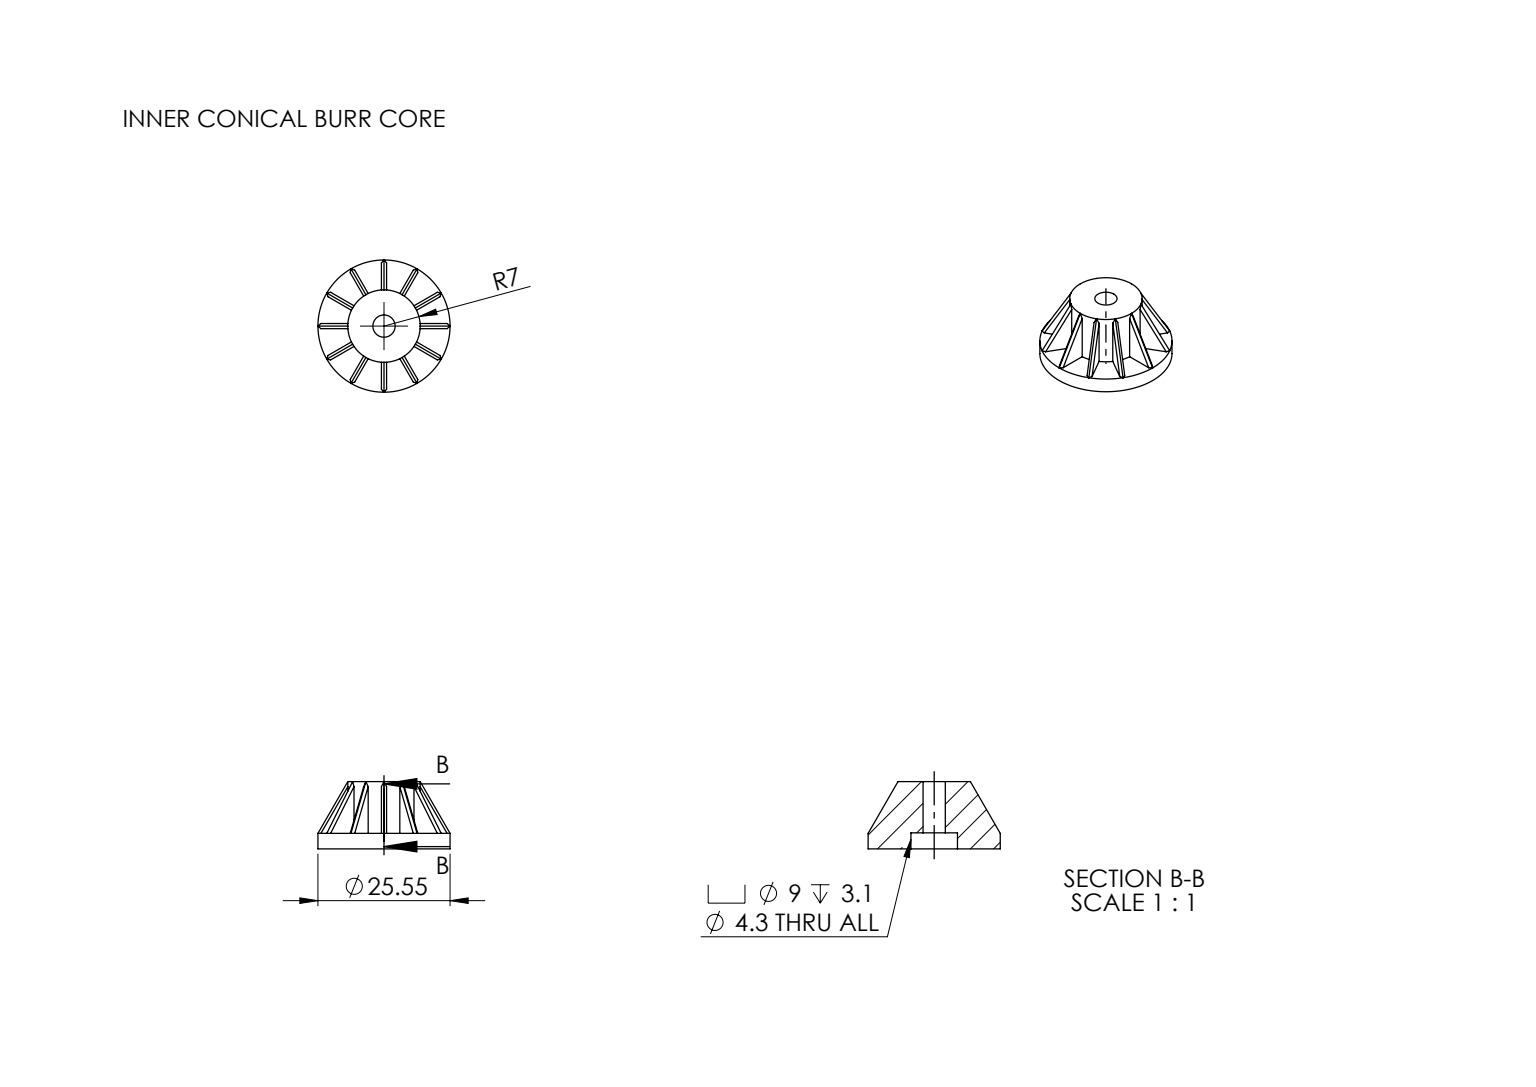
ISO-10303-21;
HEADER;
FILE_DESCRIPTION (('STEP AP214'),
    '1' );
FILE_NAME ('Inner Conical Burr Core.step',
    '2026-10-04T07:23:31',
    ( '' ),
    ( '' ),
    'SwSTEP 2.0',
    'SolidWorks 2026',
    '' );
FILE_SCHEMA (( 'AUTOMOTIVE_DESIGN' ));
ENDSEC;

DATA;
#8=VECTOR ( 'NONE', #4080, 1000.000000000000114 ) ;
#13=CARTESIAN_POINT ( 'NONE',  ( 6.296693311223917178, 19.03096903053430822, -3.058047309049999996 ) ) ;
#14=PRODUCT_DEFINITION ( 'UNKNOWN', '', #3514, #8030 ) ;
#17=EDGE_LOOP ( 'NONE', ( #5267, #4224, #10502 ) ) ;
#18=ORIENTED_EDGE ( 'NONE', *, *, #6824, .T. ) ;
#20=VERTEX_POINT ( 'NONE', #2725 ) ;
#21=DIRECTION ( 'NONE',  ( -0.000000000000000000, 1.000000000000000000, -0.000000000000000000 ) ) ;
#22=EDGE_LOOP ( 'NONE', ( #2895, #8859 ) ) ;
#23=FACE_OUTER_BOUND ( 'NONE', #10644, .T. ) ;
#26=EDGE_CURVE ( 'NONE', #5713, #6934, #4532, .T. ) ;
#34=AXIS2_PLACEMENT_3D ( 'NONE', #3449, #3389, #7599 ) ;
#41=LINE ( 'NONE', #2461, #2290 ) ;
#45=EDGE_CURVE ( 'NONE', #4079, #9358, #1978, .T. ) ;
#49=VECTOR ( 'NONE', #6901, 1000.000000000000000 ) ;
#53=LINE ( 'NONE', #1004, #7949 ) ;
#54=VECTOR ( 'NONE', #4758, 1000.000000000000000 ) ;
#62=DIRECTION ( 'NONE',  ( 0.000000000000000000, 1.000000000000000000, 0.000000000000000000 ) ) ;
#63=PLANE ( 'NONE',  #9863 ) ;
#78=CARTESIAN_POINT ( 'NONE',  ( 3.785909150703048454, 19.34316356887877220, -5.890223162633865250 ) ) ;
#89=CARTESIAN_POINT ( 'NONE',  ( 6.999999999999997335, 19.66631150450990617, 0.1668442477450632899 ) ) ;
#102=ORIENTED_EDGE ( 'NONE', *, *, #949, .F. ) ;
#115=CARTESIAN_POINT ( 'NONE',  ( 0.000000000000000000, 20.00000000000000355, 0.000000000000000000 ) ) ;
#136=CARTESIAN_POINT ( 'NONE',  ( -7.211537444790369733, 10.00000000000000355, -6.776463540776874517 ) ) ;
#144=ADVANCED_FACE ( 'NONE', ( #9538 ), #8711, .T. ) ;
#150=CYLINDRICAL_SURFACE ( 'NONE', #10591, 4.500000000000000888 ) ;
#151=DIRECTION ( 'NONE',  ( -0.8838834764831844382, -0.3535533905932726206, 0.3061862178478983454 ) ) ;
#153=AXIS2_PLACEMENT_3D ( 'NONE', #2387, #10130, #10796 ) ;
#154=CIRCLE ( 'NONE', #1379, 12.77350269189627063 ) ;
#159=CARTESIAN_POINT ( 'NONE',  ( -6.062177826491028654, 20.00000000000000355, -3.500000000000069722 ) ) ;
#162=CARTESIAN_POINT ( 'NONE',  ( -3.066987298107830995, 10.00000000000000355, 6.312177826491043753 ) ) ;
#165=CARTESIAN_POINT ( 'NONE',  ( 4.500000000000000888, 10.10000000000000497, 0.000000000000000000 ) ) ;
#173=CARTESIAN_POINT ( 'NONE',  ( 2.632990618166809235E-16, 7.000000000000003553, 2.149999999999999911 ) ) ;
#174=DIRECTION ( 'NONE',  ( 0.000000000000000000, 0.000000000000000000, 1.000000000000000000 ) ) ;
#185=DIRECTION ( 'NONE',  ( 0.000000000000000000, -1.000000000000000000, 0.000000000000000000 ) ) ;
#196=EDGE_CURVE ( 'NONE', #620, #978, #10271, .T. ) ;
#200=ORIENTED_EDGE ( 'NONE', *, *, #382, .F. ) ;
#213=ORIENTED_EDGE ( 'NONE', *, *, #10024, .F. ) ;
#219=EDGE_LOOP ( 'NONE', ( #2618, #7161, #8269, #2550 ) ) ;
#221=CARTESIAN_POINT ( 'NONE',  ( 0.000000000000000000, 7.000000000000003553, 0.000000000000000000 ) ) ;
#222=DIRECTION ( 'NONE',  ( 0.000000000000000000, 1.000000000000000000, 0.000000000000000000 ) ) ;
#244=DIRECTION ( 'NONE',  ( 0.000000000000000000, 1.000000000000000000, 0.000000000000000000 ) ) ;
#253=AXIS2_PLACEMENT_3D ( 'NONE', #6290, #1159, #5410 ) ;
#263=DIRECTION ( 'NONE',  ( 0.6546536707079723127, -0.000000000000000000, -0.7559289460184587250 ) ) ;
#276=( BOUNDED_CURVE ( )  B_SPLINE_CURVE ( 3, ( #9723, #2251, #5583, #2149 ),
 .UNSPECIFIED., .F., .F. ) 
 B_SPLINE_CURVE_WITH_KNOTS ( ( 4, 4 ),
 ( 2.284520705739658375, 2.356010155625179792 ),
 .UNSPECIFIED. ) 
 CURVE ( )  GEOMETRIC_REPRESENTATION_ITEM ( )  RATIONAL_B_SPLINE_CURVE ( ( 1.000000000000000000, 0.9995741502243209453, 0.9995741502243209453, 1.000000000000000000 ) ) 
 REPRESENTATION_ITEM ( '' )  );
#277=DIRECTION ( 'NONE',  ( -0.2500000000000041078, -0.8660254037844380415, 0.4330127018922181881 ) ) ;
#280=DIRECTION ( 'NONE',  ( -0.000000000000000000, 1.000000000000000000, -0.000000000000000000 ) ) ;
#281=CARTESIAN_POINT ( 'NONE',  ( -0.5000000000000001110, 10.00000000000000355, -6.982120021884469452 ) ) ;
#283=DIRECTION ( 'NONE',  ( 0.000000000000000000, 0.000000000000000000, 1.000000000000000000 ) ) ;
#287=PLANE ( 'NONE',  #10755 ) ;
#291=ORIENTED_EDGE ( 'NONE', *, *, #10657, .F. ) ;
#294=ORIENTED_EDGE ( 'NONE', *, *, #5471, .F. ) ;
#301=CARTESIAN_POINT ( 'NONE',  ( -5.978755702618581580, 19.66631150450990617, 3.644491357022453748 ) ) ;
#302=CARTESIAN_POINT ( 'NONE',  ( 0.2500000000000019984, 0.000000000000000000, -0.4330127018922181326 ) ) ;
#307=EDGE_CURVE ( 'NONE', #620, #1515, #1911, .T. ) ;
#308=DIRECTION ( 'NONE',  ( 0.000000000000000000, 1.000000000000000000, 0.000000000000000000 ) ) ;
#309=ADVANCED_FACE ( 'NONE', ( #3677 ), #6334, .F. ) ;
#312=CARTESIAN_POINT ( 'NONE',  ( 11.42163336986832611, 7.781088913245561400, -7.171633369868279928 ) ) ;
#320=AXIS2_PLACEMENT_3D ( 'NONE', #10601, #7911, #7226 ) ;
#324=CARTESIAN_POINT ( 'NONE',  ( -5.812177826491105037, 10.00000000000000355, 3.933012701892163676 ) ) ;
#328=AXIS2_PLACEMENT_3D ( 'NONE', #8665, #3636, #7020 ) ;
#334=( BOUNDED_CURVE ( )  B_SPLINE_CURVE ( 3, ( #9140, #1571, #4960, #8309 ),
 .UNSPECIFIED., .F., .F. ) 
 B_SPLINE_CURVE_WITH_KNOTS ( ( 4, 4 ),
 ( 2.284520705739657931, 2.356010155625178015 ),
 .UNSPECIFIED. ) 
 CURVE ( )  GEOMETRIC_REPRESENTATION_ITEM ( )  RATIONAL_B_SPLINE_CURVE ( ( 1.000000000000000000, 0.9995741502243209453, 0.9995741502243209453, 1.000000000000000000 ) ) 
 REPRESENTATION_ITEM ( '' )  );
#336=DIRECTION ( 'NONE',  ( 0.000000000000000000, 0.000000000000000000, -1.000000000000000000 ) ) ;
#340=ORIENTED_EDGE ( 'NONE', *, *, #4019, .T. ) ;
#343=CYLINDRICAL_SURFACE ( 'NONE', #9212, 12.77350269189627063 ) ;
#354=CARTESIAN_POINT ( 'NONE',  ( 6.145599950363597408, 19.66631150450990972, -3.355508642977475198 ) ) ;
#363=AXIS2_PLACEMENT_3D ( 'NONE', #7383, #10762, #7726 ) ;
#370=CARTESIAN_POINT ( 'NONE',  ( -4.336808689942017736E-16, 20.00000000000000355, 6.999999999999997335 ) ) ;
#375=VERTEX_POINT ( 'NONE', #4612 ) ;
#378=CARTESIAN_POINT ( 'NONE',  ( -7.171633369868398056, 7.781088913245559624, 11.42163336986824973 ) ) ;
#382=EDGE_CURVE ( 'NONE', #8258, #528, #7233, .T. ) ;
#384=AXIS2_PLACEMENT_3D ( 'NONE', #4121, #4890, #851 ) ;
#386=CARTESIAN_POINT ( 'NONE',  ( -5.796693311223947376, 10.00000000000000355, 3.924072712834399734 ) ) ;
#396=EDGE_CURVE ( 'NONE', #5862, #7391, #2207, .T. ) ;
#397=CIRCLE ( 'NONE', #8311, 6.999999999999997335 ) ;
#399=VERTEX_POINT ( 'NONE', #8842 ) ;
#401=CIRCLE ( 'NONE', #10807, 6.999999999999997335 ) ;
#403=CARTESIAN_POINT ( 'NONE',  ( 0.000000000000000000, 20.00000000000000355, -6.999999999999997335 ) ) ;
#417=VERTEX_POINT ( 'NONE', #2913 ) ;
#423=CARTESIAN_POINT ( 'NONE',  ( -2.857142857142858983, 10.00000000000000355, -9.474358296526935064 ) ) ;
#425=FACE_OUTER_BOUND ( 'NONE', #10415, .T. ) ;
#426=PLANE ( 'NONE',  #3198 ) ;
#428=EDGE_LOOP ( 'NONE', ( #6689, #3315, #4054 ) ) ;
#429=ORIENTED_EDGE ( 'NONE', *, *, #6271, .F. ) ;
#430=ORIENTED_EDGE ( 'NONE', *, *, #4396, .T. ) ;
#432=DIRECTION ( 'NONE',  ( -0.4999999999999919509, 0.000000000000000000, -0.8660254037844432595 ) ) ;
#438=ORIENTED_EDGE ( 'NONE', *, *, #10019, .T. ) ;
#446=EDGE_CURVE ( 'NONE', #7282, #1433, #4666, .T. ) ;
#447=CARTESIAN_POINT ( 'NONE',  ( 0.000000000000000000, 20.00000000000000355, 0.000000000000000000 ) ) ;
#453=EDGE_CURVE ( 'NONE', #3864, #1133, #3229, .T. ) ;
#462=PLANE ( 'NONE',  #6027 ) ;
#472=CARTESIAN_POINT ( 'NONE',  ( 0.000000000000000000, 20.00000000000000355, 0.000000000000000000 ) ) ;
#473=CARTESIAN_POINT ( 'NONE',  ( -6.348076211353412823, 10.00000000000000355, 11.26313972081436532 ) ) ;
#478=EDGE_CURVE ( 'NONE', #10364, #8941, #3461, .T. ) ;
#496=ORIENTED_EDGE ( 'NONE', *, *, #2584, .T. ) ;
#501=ORIENTED_EDGE ( 'NONE', *, *, #4410, .F. ) ;
#512=LINE ( 'NONE', #7202, #5833 ) ;
#523=CARTESIAN_POINT ( 'NONE',  ( 5.446152422706636465, 10.00000000000000355, -2.566987298107767490 ) ) ;
#524=ORIENTED_EDGE ( 'NONE', *, *, #1672, .T. ) ;
#525=EDGE_CURVE ( 'NONE', #5936, #10248, #7856, .T. ) ;
#526=CIRCLE ( 'NONE', #1771, 12.77350269189627063 ) ;
#528=VERTEX_POINT ( 'NONE', #281 ) ;
#531=LINE ( 'NONE', #8048, #2356 ) ;
#557=CARTESIAN_POINT ( 'NONE',  ( -6.999999999999994671, 19.66631150450992749, -0.1668442477451158867 ) ) ;
#566=AXIS2_PLACEMENT_3D ( 'NONE', #6788, #151, #987 ) ;
#567=EDGE_CURVE ( 'NONE', #9293, #10413, #10782, .T. ) ;
#569=AXIS2_PLACEMENT_3D ( 'NONE', #4292, #5896, #6784 ) ;
#570=DIRECTION ( 'NONE',  ( -1.000000000000000000, 0.000000000000000000, 0.000000000000000000 ) ) ;
#573=CARTESIAN_POINT ( 'NONE',  ( 3.058047309050023088, 10.00000000000000355, -6.296693311223907408 ) ) ;
#576=AXIS2_PLACEMENT_3D ( 'NONE', #6748, #5973, #10110 ) ;
#583=CIRCLE ( 'NONE', #4834, 6.999999999999997335 ) ;
#586=ORIENTED_EDGE ( 'NONE', *, *, #567, .T. ) ;
#588=DIRECTION ( 'NONE',  ( -1.000000000000000000, 0.000000000000000000, -1.047444401652940007E-14 ) ) ;
#592=PLANE ( 'NONE',  #2028 ) ;
#593=DIRECTION ( 'NONE',  ( -0.000000000000000000, -1.000000000000000000, -0.000000000000000000 ) ) ;
#594=DIRECTION ( 'NONE',  ( 0.000000000000000000, 1.000000000000000000, 0.000000000000000000 ) ) ;
#595=AXIS2_PLACEMENT_3D ( 'NONE', #2399, #9367, #7543 ) ;
#600=CARTESIAN_POINT ( 'NONE',  ( -3.924072712834378862, 19.03096903053431888, -5.796693311223959810 ) ) ;
#603=ORIENTED_EDGE ( 'NONE', *, *, #8062, .F. ) ;
#604=LINE ( 'NONE', #4915, #6711 ) ;
#606=LINE ( 'NONE', #10829, #1633 ) ;
#613=LINE ( 'NONE', #784, #5147 ) ;
#615=PLANE ( 'NONE',  #10718 ) ;
#617=DIRECTION ( 'NONE',  ( -0.5000000000000009992, -0.8660254037844380415, -5.237222008264710288E-15 ) ) ;
#620=VERTEX_POINT ( 'NONE', #910 ) ;
#622=ORIENTED_EDGE ( 'NONE', *, *, #2384, .T. ) ;
#623=UNCERTAINTY_MEASURE_WITH_UNIT (LENGTH_MEASURE( 1.000000000000000082E-05 ), #723, 'distance_accuracy_value', 'NONE');
#626=CARTESIAN_POINT ( 'NONE',  ( 6.296693311223917178, 10.00000000000000355, -3.058047309050000440 ) ) ;
#628=ADVANCED_FACE ( 'NONE', ( #4398 ), #5994, .T. ) ;
#639=CARTESIAN_POINT ( 'NONE',  ( -3.644491357022560329, 19.66631150450991328, 5.978755702618518519 ) ) ;
#643=ADVANCED_FACE ( 'NONE', ( #9413 ), #7049, .T. ) ;
#656=ORIENTED_EDGE ( 'NONE', *, *, #8957, .F. ) ;
#660=EDGE_LOOP ( 'NONE', ( #8805, #3492, #5444 ) ) ;
#664=VECTOR ( 'NONE', #5477, 1000.000000000000000 ) ;
#667=( NAMED_UNIT ( * ) SI_UNIT ( $, .STERADIAN. ) SOLID_ANGLE_UNIT ( ) );
#671=DIRECTION ( 'NONE',  ( -0.5000000000000009992, -0.8660254037844380415, -5.237222008264710288E-15 ) ) ;
#673=APPLICATION_CONTEXT ( 'automotive_design' ) ;
#680=( BOUNDED_CURVE ( )  B_SPLINE_CURVE ( 3, ( #1827, #826, #9316, #8327 ),
 .UNSPECIFIED., .F., .F. ) 
 B_SPLINE_CURVE_WITH_KNOTS ( ( 4, 4 ),
 ( 2.284520705739662816, 2.356010155625183344 ),
 .UNSPECIFIED. ) 
 CURVE ( )  GEOMETRIC_REPRESENTATION_ITEM ( )  RATIONAL_B_SPLINE_CURVE ( ( 1.000000000000000000, 0.9995741502243209453, 0.9995741502243209453, 1.000000000000000000 ) ) 
 REPRESENTATION_ITEM ( '' )  );
#685=FACE_OUTER_BOUND ( 'NONE', #2794, .T. ) ;
#688=EDGE_CURVE ( 'NONE', #7766, #10229, #10434, .T. ) ;
#689=VERTEX_POINT ( 'NONE', #7976 ) ;
#691=PLANE ( 'NONE',  #569 ) ;
#692=CARTESIAN_POINT ( 'NONE',  ( 5.796693311223918066, 10.00000000000000355, -3.924072712834439702 ) ) ;
#694=DIRECTION ( 'NONE',  ( 0.5000000000000009992, 0.8660254037844380415, 5.237222008264710288E-15 ) ) ;
#699=EDGE_CURVE ( 'NONE', #8354, #9358, #9835, .T. ) ;
#701=LINE ( 'NONE', #1368, #8 ) ;
#723=( LENGTH_UNIT ( ) NAMED_UNIT ( * ) SI_UNIT ( .MILLI., .METRE. ) );
#726=CARTESIAN_POINT ( 'NONE',  ( 0.000000000000000000, 10.00000000000000355, 0.000000000000000000 ) ) ;
#731=ORIENTED_EDGE ( 'NONE', *, *, #3404, .F. ) ;
#732=ORIENTED_EDGE ( 'NONE', *, *, #949, .T. ) ;
#737=LINE ( 'NONE', #6601, #10727 ) ;
#740=CARTESIAN_POINT ( 'NONE',  ( -2.850480947161592393, 19.75000000000000000, -5.937177826491103261 ) ) ;
#742=FACE_OUTER_BOUND ( 'NONE', #10182, .T. ) ;
#748=VERTEX_POINT ( 'NONE', #2062 ) ;
#757=CARTESIAN_POINT ( 'NONE',  ( 3.924072712834419718, 10.00000000000000355, 5.796693311223933165 ) ) ;
#758=AXIS2_PLACEMENT_3D ( 'NONE', #2810, #6208, #9567 ) ;
#760=ORIENTED_EDGE ( 'NONE', *, *, #1166, .T. ) ;
#761=VECTOR ( 'NONE', #8157, 1000.000000000000000 ) ;
#762=VECTOR ( 'NONE', #6178, 1000.000000000000114 ) ;
#768=LINE ( 'NONE', #8263, #2119 ) ;
#772=FACE_OUTER_BOUND ( 'NONE', #7291, .T. ) ;
#773=CARTESIAN_POINT ( 'NONE',  ( 0.000000000000000000, 7.000000000000003553, -4.500000000000000888 ) ) ;
#775=CIRCLE ( 'NONE', #8006, 6.999999999999997335 ) ;
#776=EDGE_LOOP ( 'NONE', ( #10832, #8415, #8860, #10571 ) ) ;
#777=EDGE_LOOP ( 'NONE', ( #3949, #5123, #7353, #340, #8376, #4998 ) ) ;
#784=CARTESIAN_POINT ( 'NONE',  ( -5.437177826491026877, 19.75000000000000355, -3.716506350946172876 ) ) ;
#793=ORIENTED_EDGE ( 'NONE', *, *, #8651, .F. ) ;
#797=EDGE_CURVE ( 'NONE', #6584, #9935, #4622, .T. ) ;
#801=LINE ( 'NONE', #740, #2804 ) ;
#805=PLANE ( 'NONE',  #10636 ) ;
#808=ORIENTED_EDGE ( 'NONE', *, *, #2666, .F. ) ;
#812=EDGE_CURVE ( 'NONE', #8587, #10544, #2924, .T. ) ;
#816=DIRECTION ( 'NONE',  ( 0.8838834764831839941, 0.3535533905932757293, 0.3061862178478963470 ) ) ;
#817=DIRECTION ( 'NONE',  ( 0.7559289460184611675, 0.000000000000000000, -0.6546536707079694262 ) ) ;
#818=ADVANCED_FACE ( 'NONE', ( #6639 ), #615, .F. ) ;
#819=ORIENTED_EDGE ( 'NONE', *, *, #6227, .T. ) ;
#824=VERTEX_POINT ( 'NONE', #3298 ) ;
#826=CARTESIAN_POINT ( 'NONE',  ( -3.644491357022439537, 19.66631150450991328, -5.978755702618592238 ) ) ;
#827=DIRECTION ( 'NONE',  ( -0.3061862178479081154, 0.3535533905932724541, 0.8838834764831812185 ) ) ;
#829=ORIENTED_EDGE ( 'NONE', *, *, #10797, .T. ) ;
#842=ORIENTED_EDGE ( 'NONE', *, *, #8332, .T. ) ;
#851=DIRECTION ( 'NONE',  ( 0.000000000000000000, 0.000000000000000000, 1.000000000000000000 ) ) ;
#854=FACE_OUTER_BOUND ( 'NONE', #4694, .T. ) ;
#858=ORIENTED_EDGE ( 'NONE', *, *, #9260, .F. ) ;
#863=CARTESIAN_POINT ( 'NONE',  ( 3.058047309049977791, 19.03096903053433309, 6.296693311223928724 ) ) ;
#871=LINE ( 'NONE', #3396, #9310 ) ;
#874=DIRECTION ( 'NONE',  ( -0.000000000000000000, -1.000000000000000000, -0.000000000000000000 ) ) ;
#880=VECTOR ( 'NONE', #1605, 1000.000000000000114 ) ;
#895=DIRECTION ( 'NONE',  ( -0.1767766952966370597, -0.3535533905932738419, 0.9185586535436917055 ) ) ;
#897=CYLINDRICAL_SURFACE ( 'NONE', #5644, 6.999999999999997335 ) ;
#903=DIRECTION ( 'NONE',  ( 0.000000000000000000, 0.000000000000000000, 1.000000000000000000 ) ) ;
#909=ORIENTED_EDGE ( 'NONE', *, *, #4582, .F. ) ;
#910=CARTESIAN_POINT ( 'NONE',  ( -3.500000000000049294, 20.00000000000000355, 6.062177826491040200 ) ) ;
#915=VERTEX_POINT ( 'NONE', #4880 ) ;
#925=CARTESIAN_POINT ( 'NONE',  ( 6.982120021884465899, 19.03096903053429401, 0.5000000000000244249 ) ) ;
#938=LINE ( 'NONE', #4306, #3108 ) ;
#943=CIRCLE ( 'NONE', #10817, 2.149999999999999911 ) ;
#947=AXIS2_PLACEMENT_3D ( 'NONE', #8244, #10531, #8975 ) ;
#949=EDGE_CURVE ( 'NONE', #3818, #3051, #10896, .T. ) ;
#964=VECTOR ( 'NONE', #1264, 1000.000000000000000 ) ;
#967=ORIENTED_EDGE ( 'NONE', *, *, #2281, .F. ) ;
#978=VERTEX_POINT ( 'NONE', #1668 ) ;
#979=CARTESIAN_POINT ( 'NONE',  ( 0.000000000000000000, 10.00000000000000355, 0.000000000000000000 ) ) ;
#984=( BOUNDED_CURVE ( )  B_SPLINE_CURVE ( 3, ( #8489, #6736, #6844, #2563 ),
 .UNSPECIFIED., .F., .T. ) 
 B_SPLINE_CURVE_WITH_KNOTS ( ( 4, 4 ),
 ( 3.927175151554402888, 3.998664601439924304 ),
 .UNSPECIFIED. ) 
 CURVE ( )  GEOMETRIC_REPRESENTATION_ITEM ( )  RATIONAL_B_SPLINE_CURVE ( ( 1.000000000000000000, 0.9995741502243209453, 0.9995741502243209453, 1.000000000000000000 ) ) 
 REPRESENTATION_ITEM ( '' )  );
#986=LINE ( 'NONE', #9545, #1256 ) ;
#987=DIRECTION ( 'NONE',  ( -0.4330127018922191318, 0.8660254037844380415, -0.2500000000000026090 ) ) ;
#988=DIRECTION ( 'NONE',  ( 0.4999999999999980016, 0.000000000000000000, 0.8660254037844398178 ) ) ;
#990=ORIENTED_EDGE ( 'NONE', *, *, #7446, .T. ) ;
#992=LINE ( 'NONE', #3335, #8666 ) ;
#996=ORIENTED_EDGE ( 'NONE', *, *, #453, .F. ) ;
#997=EDGE_CURVE ( 'NONE', #6764, #7282, #10390, .T. ) ;
#999=DIRECTION ( 'NONE',  ( 0.000000000000000000, -1.000000000000000000, 0.000000000000000000 ) ) ;
#1001=ADVANCED_FACE ( 'NONE', ( #1013 ), #7805, .F. ) ;
#1004=CARTESIAN_POINT ( 'NONE',  ( -11.06217782649114412, 10.00000000000000533, 6.386751345948026071 ) ) ;
#1008=EDGE_CURVE ( 'NONE', #9883, #7303, #1839, .T. ) ;
#1013=FACE_OUTER_BOUND ( 'NONE', #2172, .T. ) ;
#1016=EDGE_CURVE ( 'NONE', #8941, #10020, #1128, .T. ) ;
#1017=ORIENTED_EDGE ( 'NONE', *, *, #3787, .T. ) ;
#1019=( GEOMETRIC_REPRESENTATION_CONTEXT ( 3 ) GLOBAL_UNCERTAINTY_ASSIGNED_CONTEXT ( ( #1395 ) ) GLOBAL_UNIT_ASSIGNED_CONTEXT ( ( #2530, #3296, #4932 ) ) REPRESENTATION_CONTEXT ( 'NONE', 'WORKASPACE' ) );
#1026=CARTESIAN_POINT ( 'NONE',  ( -5.890223162633902554, 19.34316356887877220, 3.785909150702991166 ) ) ;
#1032=EDGE_LOOP ( 'NONE', ( #3309, #9854, #6146, #10751, #8965, #2173 ) ) ;
#1037=VECTOR ( 'NONE', #2963, 1000.000000000000000 ) ;
#1043=DIRECTION ( 'NONE',  ( -0.2499999999999980016, 0.8660254037844380415, -0.4330127018922217408 ) ) ;
#1049=ORIENTED_EDGE ( 'NONE', *, *, #196, .T. ) ;
#1068=DIRECTION ( 'NONE',  ( 0.000000000000000000, 0.000000000000000000, -1.000000000000000000 ) ) ;
#1069=DIRECTION ( 'NONE',  ( 0.5000000000000009992, 0.000000000000000000, -0.8660254037844380415 ) ) ;
#1071=AXIS2_PLACEMENT_3D ( 'NONE', #8171, #7438, #3226 ) ;
#1073=AXIS2_PLACEMENT_3D ( 'NONE', #10856, #9237, #8408 ) ;
#1074=ORIENTED_EDGE ( 'NONE', *, *, #3776, .T. ) ;
#1079=LINE ( 'NONE', #10349, #6951 ) ;
#1091=ORIENTED_EDGE ( 'NONE', *, *, #2592, .F. ) ;
#1092=ORIENTED_EDGE ( 'NONE', *, *, #10848, .F. ) ;
#1101=CARTESIAN_POINT ( 'NONE',  ( 0.000000000000000000, 7.000000000000003553, 0.000000000000000000 ) ) ;
#1102=FACE_OUTER_BOUND ( 'NONE', #9137, .T. ) ;
#1104=VECTOR ( 'NONE', #7309, 999.9999999999998863 ) ;
#1107=CARTESIAN_POINT ( 'NONE',  ( 0.5000000000000000000, 0.000000000000000000, 0.000000000000000000 ) ) ;
#1109=CIRCLE ( 'NONE', #2847, 6.999999999999997335 ) ;
#1112=CARTESIAN_POINT ( 'NONE',  ( 5.796693311223892309, 19.03096903053431532, 3.924072712834481447 ) ) ;
#1117=( BOUNDED_CURVE ( )  B_SPLINE_CURVE ( 3, ( #5452, #2124, #8041, #4691 ),
 .UNSPECIFIED., .F., .F. ) 
 B_SPLINE_CURVE_WITH_KNOTS ( ( 4, 4 ),
 ( 3.927175151554401999, 3.998664601439922972 ),
 .UNSPECIFIED. ) 
 CURVE ( )  GEOMETRIC_REPRESENTATION_ITEM ( )  RATIONAL_B_SPLINE_CURVE ( ( 1.000000000000000000, 0.9995741502243209453, 0.9995741502243209453, 1.000000000000000000 ) ) 
 REPRESENTATION_ITEM ( '' )  );
#1122=ORIENTED_EDGE ( 'NONE', *, *, #3481, .F. ) ;
#1128=LINE ( 'NONE', #10289, #4919 ) ;
#1129=EDGE_CURVE ( 'NONE', #9174, #2551, #4750, .T. ) ;
#1133=VERTEX_POINT ( 'NONE', #6203 ) ;
#1134=EDGE_LOOP ( 'NONE', ( #1798, #4684, #4225, #996 ) ) ;
#1137=CARTESIAN_POINT ( 'NONE',  ( 0.000000000000000000, 10.00000000000000355, 0.000000000000000000 ) ) ;
#1145=CARTESIAN_POINT ( 'NONE',  ( 3.355508642977490297, 19.66631150450992749, -6.145599950363587638 ) ) ;
#1146=PLANE ( 'NONE',  #1766 ) ;
#1147=EDGE_CURVE ( 'NONE', #10413, #5164, #4139, .T. ) ;
#1155=CARTESIAN_POINT ( 'NONE',  ( 11.92163336986827815, 7.781088913245563177, 6.305607966083920601 ) ) ;
#1159=DIRECTION ( 'NONE',  ( 0.000000000000000000, 1.000000000000000000, 0.000000000000000000 ) ) ;
#1166=EDGE_CURVE ( 'NONE', #5553, #2933, #871, .T. ) ;
#1167=EDGE_LOOP ( 'NONE', ( #7022, #430, #3791, #5634, #3288, #6183 ) ) ;
#1175=CARTESIAN_POINT ( 'NONE',  ( 6.982120021884465899, 10.00000000000000355, 0.5000000000000244249 ) ) ;
#1183=ORIENTED_EDGE ( 'NONE', *, *, #8064, .F. ) ;
#1184=ORIENTED_EDGE ( 'NONE', *, *, #1672, .F. ) ;
#1185=DIRECTION ( 'NONE',  ( 0.4330127018922207971, -0.8660254037844380415, -0.2499999999999995004 ) ) ;
#1196=EDGE_LOOP ( 'NONE', ( #731, #8937, #10125 ) ) ;
#1199=EDGE_CURVE ( 'NONE', #10020, #10364, #1818, .T. ) ;
#1206=CARTESIAN_POINT ( 'NONE',  ( -3.058047309049933382, 19.03096903053431532, -6.296693311223948264 ) ) ;
#1213=EDGE_CURVE ( 'NONE', #1851, #7784, #154, .T. ) ;
#1223=LINE ( 'NONE', #1175, #1967 ) ;
#1229=CARTESIAN_POINT ( 'NONE',  ( 0.5000000000000000000, 10.00000000000000355, -5.999999999999998224 ) ) ;
#1239=DIRECTION ( 'NONE',  ( -1.000000000000000000, 0.000000000000000000, -1.047444401652940007E-14 ) ) ;
#1241=CARTESIAN_POINT ( 'NONE',  ( 5.665063509461120361, 10.00000000000000355, -10.81217782649108372 ) ) ;
#1245=ORIENTED_EDGE ( 'NONE', *, *, #699, .T. ) ;
#1247=VERTEX_POINT ( 'NONE', #7603 ) ;
#1248=CARTESIAN_POINT ( 'NONE',  ( -3.208128317448977196, 19.34316356887881128, 6.223805082245715603 ) ) ;
#1254=DIRECTION ( 'NONE',  ( 0.8660254037844380415, 0.000000000000000000, 0.5000000000000009992 ) ) ;
#1256=VECTOR ( 'NONE', #5128, 1000.000000000000000 ) ;
#1258=ORIENTED_EDGE ( 'NONE', *, *, #525, .F. ) ;
#1260=ORIENTED_EDGE ( 'NONE', *, *, #10753, .T. ) ;
#1263=PLANE ( 'NONE',  #5478 ) ;
#1264=DIRECTION ( 'NONE',  ( 0.4999999999999949485, 0.000000000000000000, 0.8660254037844415942 ) ) ;
#1266=DIRECTION ( 'NONE',  ( 0.2500000000000009992, -0.8660254037844380415, -0.4330127018922199644 ) ) ;
#1270=EDGE_CURVE ( 'NONE', #10548, #4873, #7811, .T. ) ;
#1271=EDGE_LOOP ( 'NONE', ( #4840, #1939, #3452, #622, #4084, #2284, #2605, #5069, #10916, #10769, #1975, #6829 ) ) ;
#1279=CARTESIAN_POINT ( 'NONE',  ( -12.77350269189627241, 10.00000000000000355, -1.327078395747997636E-13 ) ) ;
#1286=ORIENTED_EDGE ( 'NONE', *, *, #997, .F. ) ;
#1300=ORIENTED_EDGE ( 'NONE', *, *, #1442, .F. ) ;
#1302=DIRECTION ( 'NONE',  ( 0.000000000000000000, 0.000000000000000000, 1.000000000000000000 ) ) ;
#1312=ORIENTED_EDGE ( 'NONE', *, *, #7953, .F. ) ;
#1319=VERTEX_POINT ( 'NONE', #6766 ) ;
#1326=ORIENTED_EDGE ( 'NONE', *, *, #10181, .F. ) ;
#1327=CARTESIAN_POINT ( 'NONE',  ( -6.296693311223937606, 10.00000000000000355, 3.058047309049956475 ) ) ;
#1333=ORIENTED_EDGE ( 'NONE', *, *, #2241, .T. ) ;
#1362=CARTESIAN_POINT ( 'NONE',  ( 0.000000000000000000, 20.00000000000000355, 0.000000000000000000 ) ) ;
#1364=DIRECTION ( 'NONE',  ( 0.000000000000000000, 0.000000000000000000, 1.000000000000000000 ) ) ;
#1368=CARTESIAN_POINT ( 'NONE',  ( -3.716506350946151116, 19.75000000000000000, 5.437177826491034871 ) ) ;
#1373=CARTESIAN_POINT ( 'NONE',  ( -0.5000000000000000000, 19.03096903053429756, 6.982120021884467675 ) ) ;
#1378=EDGE_LOOP ( 'NONE', ( #10791, #2872, #5728 ) ) ;
#1379=AXIS2_PLACEMENT_3D ( 'NONE', #4184, #10264, #5902 ) ;
#1380=EDGE_CURVE ( 'NONE', #20, #748, #2431, .T. ) ;
#1388=DIRECTION ( 'NONE',  ( 0.000000000000000000, 0.000000000000000000, 1.000000000000000000 ) ) ;
#1395=UNCERTAINTY_MEASURE_WITH_UNIT (LENGTH_MEASURE( 1.000000000000000082E-05 ), #2530, 'distance_accuracy_value', 'NONE');
#1402=CYLINDRICAL_SURFACE ( 'NONE', #8139, 6.999999999999997335 ) ;
#1403=DIRECTION ( 'NONE',  ( 0.000000000000000000, 0.000000000000000000, 1.000000000000000000 ) ) ;
#1409=ORIENTED_EDGE ( 'NONE', *, *, #10098, .F. ) ;
#1425=CARTESIAN_POINT ( 'NONE',  ( -9.474358296526972367, 10.00000000000000355, 2.857142857142765724 ) ) ;
#1433=VERTEX_POINT ( 'NONE', #4565 ) ;
#1434=EDGE_CURVE ( 'NONE', #7845, #10020, #3873, .T. ) ;
#1442=EDGE_CURVE ( 'NONE', #10157, #7784, #7920, .T. ) ;
#1444=ORIENTED_EDGE ( 'NONE', *, *, #5501, .F. ) ;
#1447=CIRCLE ( 'NONE', #4129, 12.77350269189627063 ) ;
#1451=( BOUNDED_CURVE ( )  B_SPLINE_CURVE ( 3, ( #1206, #3737, #2076, #3901 ),
 .UNSPECIFIED., .F., .F. ) 
 B_SPLINE_CURVE_WITH_KNOTS ( ( 4, 4 ),
 ( 3.927175151554405552, 3.998664601439926081 ),
 .UNSPECIFIED. ) 
 CURVE ( )  GEOMETRIC_REPRESENTATION_ITEM ( )  RATIONAL_B_SPLINE_CURVE ( ( 1.000000000000000000, 0.9995741502243209453, 0.9995741502243209453, 1.000000000000000000 ) ) 
 REPRESENTATION_ITEM ( '' )  );
#1456=LINE ( 'NONE', #324, #9119 ) ;
#1460=DIRECTION ( 'NONE',  ( -0.8660254037844345998, 0.000000000000000000, -0.5000000000000071054 ) ) ;
#1464=EDGE_CURVE ( 'NONE', #824, #4079, #8657, .T. ) ;
#1472=PLANE ( 'NONE',  #4474 ) ;
#1474=DIRECTION ( 'NONE',  ( 0.000000000000000000, -1.000000000000000000, 0.000000000000000000 ) ) ;
#1475=CARTESIAN_POINT ( 'NONE',  ( 0.000000000000000000, 10.10000000000000497, 0.000000000000000000 ) ) ;
#1478=EDGE_CURVE ( 'NONE', #4041, #7282, #3720, .T. ) ;
#1480=ORIENTED_EDGE ( 'NONE', *, *, #7319, .F. ) ;
#1484=ORIENTED_EDGE ( 'NONE', *, *, #3967, .F. ) ;
#1493=ORIENTED_EDGE ( 'NONE', *, *, #9010, .T. ) ;
#1508=CARTESIAN_POINT ( 'NONE',  ( -1.214306433183764808E-14, 10.00000000000000355, -12.77350269189627063 ) ) ;
#1510=DIRECTION ( 'NONE',  ( -0.000000000000000000, 1.000000000000000000, -0.000000000000000000 ) ) ;
#1515=VERTEX_POINT ( 'NONE', #9629 ) ;
#1516=EDGE_CURVE ( 'NONE', #399, #8258, #4076, .T. ) ;
#1517=DIRECTION ( 'NONE',  ( 0.000000000000000000, -1.000000000000000000, 0.000000000000000000 ) ) ;
#1539=ORIENTED_EDGE ( 'NONE', *, *, #1741, .T. ) ;
#1544=VECTOR ( 'NONE', #2310, 1000.000000000000000 ) ;
#1548=PRESENTATION_STYLE_ASSIGNMENT (( #5045 ) ) ;
#1551=CARTESIAN_POINT ( 'NONE',  ( -6.305607966083967675, 7.781088913245563177, 11.92163336986826216 ) ) ;
#1552=CARTESIAN_POINT ( 'NONE',  ( -5.796693311223946488, 10.00000000000000355, 3.924072712834398846 ) ) ;
#1553=CARTESIAN_POINT ( 'NONE',  ( -13.47724133595217744, 7.781088913245558736, 0.4999999999998588351 ) ) ;
#1556=ORIENTED_EDGE ( 'NONE', *, *, #2418, .T. ) ;
#1560=ORIENTED_EDGE ( 'NONE', *, *, #2792, .F. ) ;
#1562=DIRECTION ( 'NONE',  ( 0.000000000000000000, -1.000000000000000000, 0.000000000000000000 ) ) ;
#1563=CARTESIAN_POINT ( 'NONE',  ( 0.000000000000000000, 20.00000000000000355, 6.999999999999997335 ) ) ;
#1565=CARTESIAN_POINT ( 'NONE',  ( -0.4330127018922190207, 0.000000000000000000, -0.2500000000000004996 ) ) ;
#1570=ADVANCED_FACE ( 'NONE', ( #7407 ), #150, .F. ) ;
#1571=CARTESIAN_POINT ( 'NONE',  ( -6.999999999999998224, 19.66631150450992749, 0.1668442477449725569 ) ) ;
#1584=EDGE_CURVE ( 'NONE', #9550, #6584, #3570, .T. ) ;
#1596=ORIENTED_EDGE ( 'NONE', *, *, #5849, .T. ) ;
#1605=DIRECTION ( 'NONE',  ( -0.2500000000000041078, -0.8660254037844380415, 0.4330127018922182436 ) ) ;
#1606=CARTESIAN_POINT ( 'NONE',  ( 7.211537444790402596, 10.00000000000000355, 6.776463540776813232 ) ) ;
#1611=ORIENTED_EDGE ( 'NONE', *, *, #45, .F. ) ;
#1614=( BOUNDED_CURVE ( )  B_SPLINE_CURVE ( 3, ( #2179, #4004, #8915, #2280 ),
 .UNSPECIFIED., .F., .F. ) 
 B_SPLINE_CURVE_WITH_KNOTS ( ( 4, 4 ),
 ( 2.284520705739659263, 2.356010155625179348 ),
 .UNSPECIFIED. ) 
 CURVE ( )  GEOMETRIC_REPRESENTATION_ITEM ( )  RATIONAL_B_SPLINE_CURVE ( ( 1.000000000000000000, 0.9995741502243209453, 0.9995741502243209453, 1.000000000000000000 ) ) 
 REPRESENTATION_ITEM ( '' )  );
#1621=LINE ( 'NONE', #3475, #5872 ) ;
#1626=ORIENTED_EDGE ( 'NONE', *, *, #2584, .F. ) ;
#1627=VECTOR ( 'NONE', #3915, 1000.000000000000000 ) ;
#1630=VERTEX_POINT ( 'NONE', #6074 ) ;
#1633=VECTOR ( 'NONE', #10042, 1000.000000000000000 ) ;
#1635=LINE ( 'NONE', #5020, #6567 ) ;
#1636=CYLINDRICAL_SURFACE ( 'NONE', #6781, 4.500000000000000888 ) ;
#1637=CARTESIAN_POINT ( 'NONE',  ( 0.000000000000000000, 10.00000000000000355, 0.000000000000000000 ) ) ;
#1638=PLANE ( 'NONE',  #6593 ) ;
#1640=( GEOMETRIC_REPRESENTATION_CONTEXT ( 3 ) GLOBAL_UNCERTAINTY_ASSIGNED_CONTEXT ( ( #623 ) ) GLOBAL_UNIT_ASSIGNED_CONTEXT ( ( #723, #5751, #9996 ) ) REPRESENTATION_CONTEXT ( 'NONE', 'WORKASPACE' ) );
#1644=DIRECTION ( 'NONE',  ( -0.2500000000000009992, 0.8660254037844380415, 0.4330127018922199089 ) ) ;
#1647=FACE_OUTER_BOUND ( 'NONE', #4376, .T. ) ;
#1660=FACE_BOUND ( 'NONE', #22, .T. ) ;
#1662=CARTESIAN_POINT ( 'NONE',  ( -7.000000000000002665, 10.00000000000000355, 0.4999999999999267253 ) ) ;
#1665=FILL_AREA_STYLE ('',( #10894 ) ) ;
#1666=ADVANCED_FACE ( 'NONE', ( #6839 ), #5249, .T. ) ;
#1668=CARTESIAN_POINT ( 'NONE',  ( -3.058047309050066165, 19.03096903053433309, 6.296693311223885203 ) ) ;
#1670=DIRECTION ( 'NONE',  ( 0.000000000000000000, -0.000000000000000000, 1.000000000000000000 ) ) ;
#1672=EDGE_CURVE ( 'NONE', #6934, #10217, #2556, .T. ) ;
#1680=EDGE_CURVE ( 'NONE', #7784, #10524, #986, .T. ) ;
#1686=ORIENTED_EDGE ( 'NONE', *, *, #7898, .T. ) ;
#1689=ORIENTED_EDGE ( 'NONE', *, *, #8064, .T. ) ;
#1694=FACE_OUTER_BOUND ( 'NONE', #4531, .T. ) ;
#1700=ORIENTED_EDGE ( 'NONE', *, *, #2592, .T. ) ;
#1721=ORIENTED_EDGE ( 'NONE', *, *, #4770, .F. ) ;
#1740=ORIENTED_EDGE ( 'NONE', *, *, #3963, .T. ) ;
#1741=EDGE_CURVE ( 'NONE', #5725, #3717, #1451, .T. ) ;
#1743=VECTOR ( 'NONE', #9170, 1000.000000000000000 ) ;
#1747=DIRECTION ( 'NONE',  ( 0.000000000000000000, 0.000000000000000000, 1.000000000000000000 ) ) ;
#1755=ORIENTED_EDGE ( 'NONE', *, *, #5501, .T. ) ;
#1758=VECTOR ( 'NONE', #8068, 999.9999999999998863 ) ;
#1763=DIRECTION ( 'NONE',  ( 0.000000000000000000, -1.000000000000000000, 0.000000000000000000 ) ) ;
#1766=AXIS2_PLACEMENT_3D ( 'NONE', #9474, #2825, #10304 ) ;
#1767=CARTESIAN_POINT ( 'NONE',  ( 5.978755702618553158, 19.66631150450991683, -3.644491357022503930 ) ) ;
#1771=AXIS2_PLACEMENT_3D ( 'NONE', #7914, #2808, #6207 ) ;
#1773=PLANE ( 'NONE',  #8825 ) ;
#1775=DIRECTION ( 'NONE',  ( -1.000000000000000000, 0.000000000000000000, -1.047444401652940007E-14 ) ) ;
#1776=CARTESIAN_POINT ( 'NONE',  ( 0.000000000000000000, 7.000000000000003553, -2.149999999999999911 ) ) ;
#1779=CARTESIAN_POINT ( 'NONE',  ( 10.31217782649109971, 10.00000000000000355, -6.531088913245519656 ) ) ;
#1787=CARTESIAN_POINT ( 'NONE',  ( 3.058047309049977791, 19.03096903053433309, 6.296693311223928724 ) ) ;
#1788=AXIS2_PLACEMENT_3D ( 'NONE', #5383, #9670, #2052 ) ;
#1792=EDGE_LOOP ( 'NONE', ( #9713, #6544 ) ) ;
#1798=ORIENTED_EDGE ( 'NONE', *, *, #6507, .F. ) ;
#1799=ORIENTED_EDGE ( 'NONE', *, *, #10098, .T. ) ;
#1800=EDGE_LOOP ( 'NONE', ( #5256, #9523, #3633, #4040 ) ) ;
#1802=ADVANCED_FACE ( 'NONE', ( #2125 ), #7260, .T. ) ;
#1806=CARTESIAN_POINT ( 'NONE',  ( -6.531088913245408634, 10.00000000000000355, -10.31217782649116188 ) ) ;
#1808=DIRECTION ( 'NONE',  ( 0.4999999999999980016, 0.000000000000000000, 0.8660254037844398178 ) ) ;
#1813=ORIENTED_EDGE ( 'NONE', *, *, #10030, .T. ) ;
#1818=LINE ( 'NONE', #10929, #9680 ) ;
#1826=ADVANCED_FACE ( 'NONE', ( #425 ), #7213, .T. ) ;
#1827=CARTESIAN_POINT ( 'NONE',  ( -3.499999999999921840, 20.00000000000000355, -6.062177826491114807 ) ) ;
#1839=LINE ( 'NONE', #173, #7737 ) ;
#1847=CARTESIAN_POINT ( 'NONE',  ( -10.81217782649101977, 10.00000000000000355, -5.665063509461230495 ) ) ;
#1851=VERTEX_POINT ( 'NONE', #10530 ) ;
#1853=CARTESIAN_POINT ( 'NONE',  ( -6.062177826491100596, 20.00000000000000355, 3.499999999999942712 ) ) ;
#1854=LINE ( 'NONE', #5289, #5843 ) ;
#1867=EDGE_CURVE ( 'NONE', #4439, #9521, #3049, .T. ) ;
#1869=DIRECTION ( 'NONE',  ( 0.000000000000000000, 1.000000000000000000, 0.000000000000000000 ) ) ;
#1870=CARTESIAN_POINT ( 'NONE',  ( 0.2499999999999990286, 0.000000000000000000, 0.4330127018922199644 ) ) ;
#1872=ADVANCED_FACE ( 'NONE', ( #2995 ), #2940, .T. ) ;
#1880=DIRECTION ( 'NONE',  ( -0.6546536707079723127, -0.000000000000000000, 0.7559289460184587250 ) ) ;
#1883=ADVANCED_FACE ( 'NONE', ( #5502 ), #5562, .T. ) ;
#1893=CARTESIAN_POINT ( 'NONE',  ( 6.062177826491073063, 20.00000000000000355, -3.499999999999989786 ) ) ;
#1904=CARTESIAN_POINT ( 'NONE',  ( 0.000000000000000000, 0.000000000000000000, 0.000000000000000000 ) ) ;
#1911=CIRCLE ( 'NONE', #10542, 6.999999999999997335 ) ;
#1914=DIRECTION ( 'NONE',  ( 0.000000000000000000, 1.000000000000000000, 0.000000000000000000 ) ) ;
#1918=ORIENTED_EDGE ( 'NONE', *, *, #7828, .F. ) ;
#1925=ORIENTED_EDGE ( 'NONE', *, *, #5459, .F. ) ;
#1927=ORIENTED_EDGE ( 'NONE', *, *, #4733, .F. ) ;
#1928=EDGE_CURVE ( 'NONE', #4468, #7572, #3729, .T. ) ;
#1933=EDGE_LOOP ( 'NONE', ( #9853, #3773, #3245, #7484, #8511, #7424 ) ) ;
#1934=CARTESIAN_POINT ( 'NONE',  ( 0.000000000000000000, 7.000000000000003553, 12.77350269189627063 ) ) ;
#1935=LINE ( 'NONE', #2084, #964 ) ;
#1938=EDGE_CURVE ( 'NONE', #9084, #4561, #9589, .T. ) ;
#1939=ORIENTED_EDGE ( 'NONE', *, *, #9085, .T. ) ;
#1949=DIRECTION ( 'NONE',  ( 0.000000000000000000, 0.000000000000000000, 1.000000000000000000 ) ) ;
#1967=VECTOR ( 'NONE', #5378, 1000.000000000000000 ) ;
#1975=ORIENTED_EDGE ( 'NONE', *, *, #9810, .T. ) ;
#1977=VECTOR ( 'NONE', #9787, 1000.000000000000114 ) ;
#1978=LINE ( 'NONE', #7770, #4195 ) ;
#1981=PLANE ( 'NONE',  #3197 ) ;
#1984=DIRECTION ( 'NONE',  ( 0.5000000000000101030, 0.000000000000000000, -0.8660254037844328234 ) ) ;
#1987=VERTEX_POINT ( 'NONE', #1241 ) ;
#1989=ORIENTED_EDGE ( 'NONE', *, *, #8416, .F. ) ;
#2006=ORIENTED_EDGE ( 'NONE', *, *, #699, .F. ) ;
#2026=DIRECTION ( 'NONE',  ( 0.000000000000000000, -1.000000000000000000, 0.000000000000000000 ) ) ;
#2028=AXIS2_PLACEMENT_3D ( 'NONE', #6557, #8003, #8927 ) ;
#2029=EDGE_CURVE ( 'NONE', #8291, #4468, #5329, .T. ) ;
#2036=CARTESIAN_POINT ( 'NONE',  ( -0.2500000000000050515, 0.000000000000000000, 0.4330127018922164117 ) ) ;
#2040=ORIENTED_EDGE ( 'NONE', *, *, #1867, .F. ) ;
#2045=CARTESIAN_POINT ( 'NONE',  ( 3.499999999999963141, 20.00000000000000355, 6.062177826491089050 ) ) ;
#2050=CARTESIAN_POINT ( 'NONE',  ( 6.062177826491051746, 20.00000000000000355, 3.500000000000027089 ) ) ;
#2052=DIRECTION ( 'NONE',  ( 0.000000000000000000, 0.000000000000000000, 1.000000000000000000 ) ) ;
#2053=LINE ( 'NONE', #1229, #4493 ) ;
#2059=ADVANCED_FACE ( 'NONE', ( #5551 ), #3998, .T. ) ;
#2062=CARTESIAN_POINT ( 'NONE',  ( -6.982120021884462346, 10.00000000000000355, -0.5000000000000731637 ) ) ;
#2063=DIRECTION ( 'NONE',  ( -0.8660254037844345998, 0.000000000000000000, -0.5000000000000071054 ) ) ;
#2074=DIRECTION ( 'NONE',  ( -0.9819805060619662962, 0.000000000000000000, 0.1889822365046104902 ) ) ;
#2075=AXIS2_PLACEMENT_3D ( 'NONE', #979, #1914, #2552 ) ;
#2076=CARTESIAN_POINT ( 'NONE',  ( -3.355508642977407252, 19.66631150450991683, -6.145599950363634711 ) ) ;
#2081=AXIS2_PLACEMENT_3D ( 'NONE', #8524, #5234, #7701 ) ;
#2083=CARTESIAN_POINT ( 'NONE',  ( 0.2499999999999960032, 0.000000000000000000, 0.4330127018922216298 ) ) ;
#2084=CARTESIAN_POINT ( 'NONE',  ( 2.566987298107748394, 10.00000000000000355, 5.446152422706646234 ) ) ;
#2086=EDGE_CURVE ( 'NONE', #1433, #8512, #6482, .T. ) ;
#2110=DIRECTION ( 'NONE',  ( -0.2500000000000009992, 0.8660254037844380415, 0.4330127018922199644 ) ) ;
#2113=VECTOR ( 'NONE', #10837, 1000.000000000000000 ) ;
#2119=VECTOR ( 'NONE', #9055, 999.9999999999998863 ) ;
#2124=CARTESIAN_POINT ( 'NONE',  ( 5.890223162633852816, 19.34316356887877930, 3.785909150703072434 ) ) ;
#2125=FACE_OUTER_BOUND ( 'NONE', #17, .T. ) ;
#2131=ORIENTED_EDGE ( 'NONE', *, *, #812, .F. ) ;
#2137=DIRECTION ( 'NONE',  ( 0.7071067811865519026, -0.3535533905932723431, 0.6123724356957903625 ) ) ;
#2138=EDGE_CURVE ( 'NONE', #2551, #2855, #512, .T. ) ;
#2143=DIRECTION ( 'NONE',  ( -0.000000000000000000, -1.000000000000000000, -0.000000000000000000 ) ) ;
#2149=CARTESIAN_POINT ( 'NONE',  ( 6.982120021884469452, 19.03096903053430466, -0.4999999999999756306 ) ) ;
#2151=VECTOR ( 'NONE', #8985, 1000.000000000000114 ) ;
#2152=ORIENTED_EDGE ( 'NONE', *, *, #7594, .T. ) ;
#2168=AXIS2_PLACEMENT_3D ( 'NONE', #3642, #8826, #10385 ) ;
#2172=EDGE_LOOP ( 'NONE', ( #8948, #4762, #2758, #10112 ) ) ;
#2173=ORIENTED_EDGE ( 'NONE', *, *, #4841, .T. ) ;
#2179=CARTESIAN_POINT ( 'NONE',  ( 3.499999999999963141, 20.00000000000000355, 6.062177826491089050 ) ) ;
#2180=VECTOR ( 'NONE', #1880, 1000.000000000000114 ) ;
#2184=PLANE ( 'NONE',  #9899 ) ;
#2194=CARTESIAN_POINT ( 'NONE',  ( 7.171633369868314567, 7.781088913245556071, -11.42163336986829236 ) ) ;
#2195=CARTESIAN_POINT ( 'NONE',  ( -10.81217782649114589, 10.00000000000000355, 5.665063509461009339 ) ) ;
#2197=ORIENTED_EDGE ( 'NONE', *, *, #6530, .T. ) ;
#2207=LINE ( 'NONE', #3021, #1037 ) ;
#2217=DIRECTION ( 'NONE',  ( -0.8660254037844415942, 0.000000000000000000, 0.4999999999999949485 ) ) ;
#2222=ORIENTED_EDGE ( 'NONE', *, *, #396, .T. ) ;
#2230=DIRECTION ( 'NONE',  ( -0.000000000000000000, 1.000000000000000000, -0.000000000000000000 ) ) ;
#2233=EDGE_LOOP ( 'NONE', ( #6255, #760, #10474, #8058, #10141, #1312 ) ) ;
#2237=DIRECTION ( 'NONE',  ( 0.000000000000000000, 0.000000000000000000, -1.000000000000000000 ) ) ;
#2238=CARTESIAN_POINT ( 'NONE',  ( 3.066987298107787030, 10.00000000000000355, -6.312177826491064181 ) ) ;
#2241=EDGE_CURVE ( 'NONE', #5566, #8414, #4050, .T. ) ;
#2248=PLANE ( 'NONE',  #363 ) ;
#2251=CARTESIAN_POINT ( 'NONE',  ( 6.999999999999998224, 19.66631150450992038, -0.1668442477450155503 ) ) ;
#2259=ADVANCED_FACE ( 'NONE', ( #9274 ), #897, .T. ) ;
#2266=CARTESIAN_POINT ( 'NONE',  ( -5.796693311223863887, 19.03096903053432598, -3.924072712834521415 ) ) ;
#2269=CARTESIAN_POINT ( 'NONE',  ( -11.06217782649100911, 10.00000000000000533, -6.386751345948263214 ) ) ;
#2279=CARTESIAN_POINT ( 'NONE',  ( -2.566987298107710203, 10.00000000000000355, -5.446152422706663998 ) ) ;
#2280=CARTESIAN_POINT ( 'NONE',  ( 3.924072712834419718, 19.03096903053430466, 5.796693311223933165 ) ) ;
#2281=EDGE_CURVE ( 'NONE', #4561, #4862, #2379, .T. ) ;
#2284=ORIENTED_EDGE ( 'NONE', *, *, #307, .T. ) ;
#2290=VECTOR ( 'NONE', #5847, 1000.000000000000000 ) ;
#2291=VECTOR ( 'NONE', #8076, 1000.000000000000000 ) ;
#2299=CARTESIAN_POINT ( 'NONE',  ( 0.5000000000000000000, 10.00000000000000355, 12.19615242270663735 ) ) ;
#2304=CARTESIAN_POINT ( 'NONE',  ( 0.5000000000000000000, 7.781088913245555183, 13.47724133595216500 ) ) ;
#2310=DIRECTION ( 'NONE',  ( -0.000000000000000000, -1.000000000000000000, -0.000000000000000000 ) ) ;
#2313=AXIS2_PLACEMENT_3D ( 'NONE', #302, #9475, #4574 ) ;
#2314=ORIENTED_EDGE ( 'NONE', *, *, #10753, .F. ) ;
#2319=CARTESIAN_POINT ( 'NONE',  ( 0.5000000000000000000, 19.03096903053429756, -6.982120021884467675 ) ) ;
#2324=CARTESIAN_POINT ( 'NONE',  ( -6.386751345947996761, 10.00000000000000533, -11.06217782649116366 ) ) ;
#2325=CARTESIAN_POINT ( 'NONE',  ( -0.2500000000000019984, 0.000000000000000000, 0.4330127018922181326 ) ) ;
#2329=AXIS2_PLACEMENT_3D ( 'NONE', #6961, #9486, #10319 ) ;
#2330=ADVANCED_FACE ( 'NONE', ( #2534 ), #63, .T. ) ;
#2338=CARTESIAN_POINT ( 'NONE',  ( 0.1668442477450440553, 19.66631150450991328, 6.999999999999995559 ) ) ;
#2349=ORIENTED_EDGE ( 'NONE', *, *, #3770, .T. ) ;
#2356=VECTOR ( 'NONE', #4747, 1000.000000000000000 ) ;
#2360=LINE ( 'NONE', #9096, #3479 ) ;
#2362=ORIENTED_EDGE ( 'NONE', *, *, #8396, .F. ) ;
#2370=EDGE_LOOP ( 'NONE', ( #7120, #9792, #2415, #10886, #8188, #8605 ) ) ;
#2379=LINE ( 'NONE', #9172, #6360 ) ;
#2384=EDGE_CURVE ( 'NONE', #10229, #10544, #9701, .T. ) ;
#2387=CARTESIAN_POINT ( 'NONE',  ( 0.000000000000000000, 20.00000000000000355, 0.000000000000000000 ) ) ;
#2394=EDGE_LOOP ( 'NONE', ( #7239, #5641, #7553 ) ) ;
#2395=EDGE_CURVE ( 'NONE', #375, #8941, #5120, .T. ) ;
#2397=CARTESIAN_POINT ( 'NONE',  ( 12.77350269189627063, 10.00000000000000355, 3.295974604355932848E-14 ) ) ;
#2399=CARTESIAN_POINT ( 'NONE',  ( -0.4330127018922225735, 0.000000000000000000, 0.2499999999999944766 ) ) ;
#2405=DIRECTION ( 'NONE',  ( 0.000000000000000000, 1.000000000000000000, 0.000000000000000000 ) ) ;
#2415=ORIENTED_EDGE ( 'NONE', *, *, #3422, .T. ) ;
#2416=ORIENTED_EDGE ( 'NONE', *, *, #3776, .F. ) ;
#2418=EDGE_CURVE ( 'NONE', #978, #8026, #9115, .T. ) ;
#2423=VERTEX_POINT ( 'NONE', #2427 ) ;
#2424=CARTESIAN_POINT ( 'NONE',  ( 0.3335819196118703922, 19.34316356887877220, -6.994037468151971026 ) ) ;
#2427=CARTESIAN_POINT ( 'NONE',  ( -3.924072712834379750, 10.00000000000000355, -5.796693311223960698 ) ) ;
#2428=LINE ( 'NONE', #5924, #3178 ) ;
#2431=CIRCLE ( 'NONE', #4592, 6.999999999999997335 ) ;
#2454=AXIS2_PLACEMENT_3D ( 'NONE', #10841, #6640, #4936 ) ;
#2461=CARTESIAN_POINT ( 'NONE',  ( -4.946152422706591167, 10.00000000000000355, -3.433012701892276475 ) ) ;
#2467=AXIS2_PLACEMENT_3D ( 'NONE', #2325, #10679, #8910 ) ;
#2485=VECTOR ( 'NONE', #10339, 1000.000000000000000 ) ;
#2490=ORIENTED_EDGE ( 'NONE', *, *, #9451, .T. ) ;
#2494=ORIENTED_EDGE ( 'NONE', *, *, #8332, .F. ) ;
#2498=VECTOR ( 'NONE', #6948, 1000.000000000000114 ) ;
#2499=CARTESIAN_POINT ( 'NONE',  ( 0.000000000000000000, 20.00000000000000355, 0.000000000000000000 ) ) ;
#2506=AXIS2_PLACEMENT_3D ( 'NONE', #9860, #593, #2237 ) ;
#2513=CARTESIAN_POINT ( 'NONE',  ( 6.999999999999997335, 20.00000000000000355, 2.444036937190192402E-14 ) ) ;
#2530=( LENGTH_UNIT ( ) NAMED_UNIT ( * ) SI_UNIT ( .MILLI., .METRE. ) );
#2534=FACE_OUTER_BOUND ( 'NONE', #2370, .T. ) ;
#2542=LINE ( 'NONE', #8296, #3113 ) ;
#2545=CARTESIAN_POINT ( 'NONE',  ( -6.296693311223937606, 19.03096903053434019, 3.058047309049956031 ) ) ;
#2548=ORIENTED_EDGE ( 'NONE', *, *, #5914, .T. ) ;
#2550=ORIENTED_EDGE ( 'NONE', *, *, #6336, .T. ) ;
#2551=VERTEX_POINT ( 'NONE', #9288 ) ;
#2552=DIRECTION ( 'NONE',  ( 0.000000000000000000, -0.000000000000000000, 1.000000000000000000 ) ) ;
#2554=CARTESIAN_POINT ( 'NONE',  ( -5.665063509461194968, 10.00000000000000355, 10.81217782649104109 ) ) ;
#2556=LINE ( 'NONE', #6179, #10059 ) ;
#2558=ORIENTED_EDGE ( 'NONE', *, *, #812, .T. ) ;
#2563=CARTESIAN_POINT ( 'NONE',  ( 0.000000000000000000, 20.00000000000000355, 6.999999999999997335 ) ) ;
#2573=EDGE_CURVE ( 'NONE', #5761, #5725, #801, .T. ) ;
#2577=ORIENTED_EDGE ( 'NONE', *, *, #5050, .F. ) ;
#2582=CARTESIAN_POINT ( 'NONE',  ( 0.000000000000000000, 10.00000000000000355, 0.000000000000000000 ) ) ;
#2584=EDGE_CURVE ( 'NONE', #10364, #9293, #7829, .T. ) ;
#2586=ADVANCED_FACE ( 'NONE', ( #4950 ), #7478, .T. ) ;
#2592=EDGE_CURVE ( 'NONE', #10544, #6448, #8165, .T. ) ;
#2595=CARTESIAN_POINT ( 'NONE',  ( 5.510910596163089556E-16, 7.000000000000003553, 4.500000000000000888 ) ) ;
#2603=ADVANCED_FACE ( 'NONE', ( #3667 ), #1146, .F. ) ;
#2605=ORIENTED_EDGE ( 'NONE', *, *, #7016, .T. ) ;
#2606=VERTEX_POINT ( 'NONE', #5235 ) ;
#2614=CARTESIAN_POINT ( 'NONE',  ( -0.5000000000000000000, 10.00000000000000355, 12.19615242270663202 ) ) ;
#2616=CARTESIAN_POINT ( 'NONE',  ( -12.92820323027551765, 10.00000000000000355, 0.1339745962154219039 ) ) ;
#2618=ORIENTED_EDGE ( 'NONE', *, *, #3422, .F. ) ;
#2630=AXIS2_PLACEMENT_3D ( 'NONE', #4552, #2143, #336 ) ;
#2633=DIRECTION ( 'NONE',  ( 0.000000000000000000, 1.000000000000000000, 0.000000000000000000 ) ) ;
#2634=PLANE ( 'NONE',  #576 ) ;
#2642=DIRECTION ( 'NONE',  ( 0.000000000000000000, 1.000000000000000000, 0.000000000000000000 ) ) ;
#2664=CIRCLE ( 'NONE', #7430, 6.999999999999997335 ) ;
#2666=EDGE_CURVE ( 'NONE', #8512, #4041, #2869, .T. ) ;
#2668=CARTESIAN_POINT ( 'NONE',  ( 0.000000000000000000, 10.00000000000000355, 0.000000000000000000 ) ) ;
#2670=DIRECTION ( 'NONE',  ( -0.000000000000000000, -1.000000000000000000, -0.000000000000000000 ) ) ;
#2671=PLANE ( 'NONE',  #253 ) ;
#2672=VECTOR ( 'NONE', #5836, 1000.000000000000000 ) ;
#2674=DIRECTION ( 'NONE',  ( 1.000000000000000000, 0.000000000000000000, 3.491481338843133355E-15 ) ) ;
#2675=DIRECTION ( 'NONE',  ( -0.7071067811865519026, -0.3535533905932723431, -0.6123724356957903625 ) ) ;
#2688=CARTESIAN_POINT ( 'NONE',  ( -6.223805082245704945, 19.34316356887878996, -3.208128317448997180 ) ) ;
#2689=VECTOR ( 'NONE', #8361, 1000.000000000000000 ) ;
#2690=DIRECTION ( 'NONE',  ( 0.000000000000000000, 1.000000000000000000, 0.000000000000000000 ) ) ;
#2692=CARTESIAN_POINT ( 'NONE',  ( 0.000000000000000000, 10.00000000000000355, 0.000000000000000000 ) ) ;
#2699=LINE ( 'NONE', #6981, #2485 ) ;
#2705=VECTOR ( 'NONE', #263, 1000.000000000000114 ) ;
#2720=ORIENTED_EDGE ( 'NONE', *, *, #8416, .T. ) ;
#2723=ORIENTED_EDGE ( 'NONE', *, *, #4529, .F. ) ;
#2724=ORIENTED_EDGE ( 'NONE', *, *, #10033, .F. ) ;
#2725=CARTESIAN_POINT ( 'NONE',  ( -6.296693311223874545, 10.00000000000000355, -3.058047309050087925 ) ) ;
#2726=ADVANCED_FACE ( 'NONE', ( #3943 ), #9734, .T. ) ;
#2730=DIRECTION ( 'NONE',  ( 0.8660254037844397068, 0.000000000000000000, -0.4999999999999979461 ) ) ;
#2737=ADVANCED_FACE ( 'NONE', ( #3830 ), #4623, .F. ) ;
#2743=LINE ( 'NONE', #7854, #2180 ) ;
#2744=DIRECTION ( 'NONE',  ( -0.000000000000000000, 1.000000000000000000, -0.000000000000000000 ) ) ;
#2748=EDGE_CURVE ( 'NONE', #6448, #9593, #9636, .T. ) ;
#2749=CARTESIAN_POINT ( 'NONE',  ( -3.058047309049932938, 10.00000000000000355, -6.296693311223948264 ) ) ;
#2754=DIRECTION ( 'NONE',  ( -0.000000000000000000, 1.000000000000000000, -0.000000000000000000 ) ) ;
#2755=CARTESIAN_POINT ( 'NONE',  ( -6.296693311223937606, 10.00000000000000355, 3.058047309049956031 ) ) ;
#2758=ORIENTED_EDGE ( 'NONE', *, *, #5514, .F. ) ;
#2759=ADVANCED_FACE ( 'NONE', ( #8185 ), #9836, .F. ) ;
#2773=ORIENTED_EDGE ( 'NONE', *, *, #4163, .T. ) ;
#2775=VECTOR ( 'NONE', #7477, 1000.000000000000000 ) ;
#2779=ORIENTED_EDGE ( 'NONE', *, *, #5251, .T. ) ;
#2781=FACE_OUTER_BOUND ( 'NONE', #2233, .T. ) ;
#2787=VERTEX_POINT ( 'NONE', #9785 ) ;
#2791=DIRECTION ( 'NONE',  ( 0.000000000000000000, -1.000000000000000000, 0.000000000000000000 ) ) ;
#2792=EDGE_CURVE ( 'NONE', #417, #7784, #6480, .T. ) ;
#2794=EDGE_LOOP ( 'NONE', ( #8316, #2222, #2779 ) ) ;
#2801=ORIENTED_EDGE ( 'NONE', *, *, #4682, .T. ) ;
#2804=VECTOR ( 'NONE', #7583, 999.9999999999998863 ) ;
#2808=DIRECTION ( 'NONE',  ( 0.000000000000000000, 1.000000000000000000, 0.000000000000000000 ) ) ;
#2810=CARTESIAN_POINT ( 'NONE',  ( 0.000000000000000000, 10.00000000000000355, 0.000000000000000000 ) ) ;
#2814=ADVANCED_FACE ( 'NONE', ( #4542 ), #3687, .T. ) ;
#2819=DIRECTION ( 'NONE',  ( 0.1889822365046095465, -0.000000000000000000, 0.9819805060619665182 ) ) ;
#2823=CARTESIAN_POINT ( 'NONE',  ( 0.000000000000000000, 10.00000000000000355, 0.000000000000000000 ) ) ;
#2825=DIRECTION ( 'NONE',  ( 0.8838834764831863255, -0.3535533905932720100, -0.3061862178478936269 ) ) ;
#2828=CARTESIAN_POINT ( 'NONE',  ( -3.933012701892143692, 10.00000000000000355, -5.812177826491118360 ) ) ;
#2834=CARTESIAN_POINT ( 'NONE',  ( 0.000000000000000000, 7.000000000000003553, 0.000000000000000000 ) ) ;
#2838=FACE_OUTER_BOUND ( 'NONE', #5537, .T. ) ;
#2847=AXIS2_PLACEMENT_3D ( 'NONE', #9889, #2642, #3749 ) ;
#2849=PLANE ( 'NONE',  #5816 ) ;
#2851=CARTESIAN_POINT ( 'NONE',  ( -5.665063509460962266, 10.00000000000000355, -10.81217782649115122 ) ) ;
#2855=VERTEX_POINT ( 'NONE', #9065 ) ;
#2863=DIRECTION ( 'NONE',  ( -0.6546536707079774198, 0.000000000000000000, -0.7559289460184541731 ) ) ;
#2869=( BOUNDED_CURVE ( )  B_SPLINE_CURVE ( 3, ( #7760, #4573, #354, #6113 ),
 .UNSPECIFIED., .F., .F. ) 
 B_SPLINE_CURVE_WITH_KNOTS ( ( 4, 4 ),
 ( 3.927175151554400223, 3.998664601439921640 ),
 .UNSPECIFIED. ) 
 CURVE ( )  GEOMETRIC_REPRESENTATION_ITEM ( )  RATIONAL_B_SPLINE_CURVE ( ( 1.000000000000000000, 0.9995741502243209453, 0.9995741502243209453, 1.000000000000000000 ) ) 
 REPRESENTATION_ITEM ( '' )  );
#2870=MECHANICAL_DESIGN_GEOMETRIC_PRESENTATION_REPRESENTATION('',(#5521),#1640);
#2872=ORIENTED_EDGE ( 'NONE', *, *, #2573, .T. ) ;
#2873=EDGE_CURVE ( 'NONE', #1851, #5761, #7455, .T. ) ;
#2887=CARTESIAN_POINT ( 'NONE',  ( 0.000000000000000000, 20.00000000000000355, 0.000000000000000000 ) ) ;
#2895=ORIENTED_EDGE ( 'NONE', *, *, #3220, .F. ) ;
#2896=PRODUCT_DEFINITION_SHAPE ( 'NONE', 'NONE',  #14 ) ;
#2897=DIRECTION ( 'NONE',  ( -0.7559289460184582810, 0.000000000000000000, 0.6546536707079726458 ) ) ;
#2898=DIRECTION ( 'NONE',  ( -0.8660254037844432595, 0.000000000000000000, 0.4999999999999919509 ) ) ;
#2899=CARTESIAN_POINT ( 'NONE',  ( -6.982120021884462346, 19.03096903053432243, -0.5000000000000731637 ) ) ;
#2901=DIRECTION ( 'NONE',  ( 0.000000000000000000, 0.000000000000000000, 1.000000000000000000 ) ) ;
#2902=EDGE_LOOP ( 'NONE', ( #2577, #5014, #4778, #990 ) ) ;
#2907=CARTESIAN_POINT ( 'NONE',  ( 6.223805082245728038, 19.34316356887878285, 3.208128317448950551 ) ) ;
#2908=ORIENTED_EDGE ( 'NONE', *, *, #6868, .F. ) ;
#2913=CARTESIAN_POINT ( 'NONE',  ( -6.062177826491028654, 20.00000000000000355, -3.500000000000069722 ) ) ;
#2924=( BOUNDED_CURVE ( )  B_SPLINE_CURVE ( 3, ( #4047, #8346, #5651, #9946 ),
 .UNSPECIFIED., .F., .F. ) 
 B_SPLINE_CURVE_WITH_KNOTS ( ( 4, 4 ),
 ( 3.927175151554404664, 3.998664601439924748 ),
 .UNSPECIFIED. ) 
 CURVE ( )  GEOMETRIC_REPRESENTATION_ITEM ( )  RATIONAL_B_SPLINE_CURVE ( ( 1.000000000000000000, 0.9995741502243209453, 0.9995741502243209453, 1.000000000000000000 ) ) 
 REPRESENTATION_ITEM ( '' )  );
#2926=DIRECTION ( 'NONE',  ( -0.5000000000000009992, 0.8660254037844380415, -1.745740669421570228E-15 ) ) ;
#2930=EDGE_LOOP ( 'NONE', ( #9824, #2494, #5538, #1927 ) ) ;
#2933=VERTEX_POINT ( 'NONE', #4984 ) ;
#2936=CARTESIAN_POINT ( 'NONE',  ( 0.000000000000000000, 20.00000000000000355, 0.000000000000000000 ) ) ;
#2939=FACE_OUTER_BOUND ( 'NONE', #7223, .T. ) ;
#2940=CYLINDRICAL_SURFACE ( 'NONE', #7785, 6.999999999999997335 ) ;
#2947=LINE ( 'NONE', #7217, #10623 ) ;
#2949=LINE ( 'NONE', #7219, #7293 ) ;
#2963=DIRECTION ( 'NONE',  ( 0.000000000000000000, 0.8660254037844380415, -0.5000000000000009992 ) ) ;
#2965=VERTEX_POINT ( 'NONE', #5700 ) ;
#2966=ORIENTED_EDGE ( 'NONE', *, *, #1680, .T. ) ;
#2981=ORIENTED_EDGE ( 'NONE', *, *, #8651, .T. ) ;
#2995=FACE_OUTER_BOUND ( 'NONE', #5402, .T. ) ;
#2996=CARTESIAN_POINT ( 'NONE',  ( -3.058047309050066165, 10.00000000000000355, 6.296693311223885203 ) ) ;
#2997=AXIS2_PLACEMENT_3D ( 'NONE', #10423, #8870, #6242 ) ;
#2998=VECTOR ( 'NONE', #7666, 1000.000000000000000 ) ;
#3000=ORIENTED_EDGE ( 'NONE', *, *, #5404, .T. ) ;
#3003=EDGE_CURVE ( 'NONE', #10544, #8354, #53, .T. ) ;
#3004=DIRECTION ( 'NONE',  ( 0.8660254037844363761, 0.000000000000000000, 0.5000000000000039968 ) ) ;
#3006=FACE_OUTER_BOUND ( 'NONE', #6313, .T. ) ;
#3010=VECTOR ( 'NONE', #8186, 1000.000000000000000 ) ;
#3016=CYLINDRICAL_SURFACE ( 'NONE', #1788, 6.999999999999997335 ) ;
#3019=ORIENTED_EDGE ( 'NONE', *, *, #2384, .F. ) ;
#3021=CARTESIAN_POINT ( 'NONE',  ( -0.5000000000000000000, 19.74999999999999645, 6.566987298107768822 ) ) ;
#3022=AXIS2_PLACEMENT_3D ( 'NONE', #10322, #1869, #5412 ) ;
#3024=ORIENTED_EDGE ( 'NONE', *, *, #9227, .F. ) ;
#3025=VECTOR ( 'NONE', #6122, 999.9999999999998863 ) ;
#3026=ORIENTED_EDGE ( 'NONE', *, *, #9765, .T. ) ;
#3030=VECTOR ( 'NONE', #5335, 1000.000000000000114 ) ;
#3035=DIRECTION ( 'NONE',  ( -0.5000000000000069944, 0.000000000000000000, 0.8660254037844344888 ) ) ;
#3049=LINE ( 'NONE', #9650, #9000 ) ;
#3050=DIRECTION ( 'NONE',  ( 0.000000000000000000, 0.000000000000000000, 1.000000000000000000 ) ) ;
#3051=VERTEX_POINT ( 'NONE', #10280 ) ;
#3053=ORIENTED_EDGE ( 'NONE', *, *, #1199, .F. ) ;
#3057=FACE_OUTER_BOUND ( 'NONE', #7326, .T. ) ;
#3065=ORIENTED_EDGE ( 'NONE', *, *, #5471, .T. ) ;
#3075=DIRECTION ( 'NONE',  ( 0.4330127018922226290, 0.8660254037844380415, -0.2499999999999965028 ) ) ;
#3088=FACE_OUTER_BOUND ( 'NONE', #5636, .T. ) ;
#3097=CARTESIAN_POINT ( 'NONE',  ( 0.000000000000000000, 10.00000000000000355, 0.000000000000000000 ) ) ;
#3102=EDGE_LOOP ( 'NONE', ( #5975, #4471, #7632, #808 ) ) ;
#3108=VECTOR ( 'NONE', #9442, 1000.000000000000000 ) ;
#3109=VECTOR ( 'NONE', #7730, 1000.000000000000000 ) ;
#3111=ADVANCED_FACE ( 'NONE', ( #1660, #7561 ), #1773, .F. ) ;
#3113=VECTOR ( 'NONE', #9287, 1000.000000000000000 ) ;
#3136=DIRECTION ( 'NONE',  ( 0.000000000000000000, 1.000000000000000000, 0.000000000000000000 ) ) ;
#3137=DIRECTION ( 'NONE',  ( 0.000000000000000000, -0.8660254037844380415, -0.5000000000000009992 ) ) ;
#3156=EDGE_LOOP ( 'NONE', ( #1300, #10687, #8946, #10428 ) ) ;
#3157=VERTEX_POINT ( 'NONE', #7029 ) ;
#3162=AXIS2_PLACEMENT_3D ( 'NONE', #6257, #5422, #283 ) ;
#3178=VECTOR ( 'NONE', #3137, 1000.000000000000000 ) ;
#3186=( NAMED_UNIT ( * ) PLANE_ANGLE_UNIT ( ) SI_UNIT ( $, .RADIAN. ) );
#3195=ORIENTED_EDGE ( 'NONE', *, *, #7269, .F. ) ;
#3197=AXIS2_PLACEMENT_3D ( 'NONE', #7115, #1808, #2730 ) ;
#3198=AXIS2_PLACEMENT_3D ( 'NONE', #6243, #10483, #4588 ) ;
#3199=EDGE_CURVE ( 'NONE', #9935, #9550, #1223, .T. ) ;
#3203=VECTOR ( 'NONE', #7335, 1000.000000000000114 ) ;
#3204=CARTESIAN_POINT ( 'NONE',  ( 0.5000000000000000000, 10.00000000000000355, -12.19615242270663202 ) ) ;
#3205=VECTOR ( 'NONE', #3499, 1000.000000000000227 ) ;
#3207=DIRECTION ( 'NONE',  ( 0.8660254037844380415, 0.000000000000000000, 0.5000000000000009992 ) ) ;
#3220=EDGE_CURVE ( 'NONE', #10062, #7303, #7406, .T. ) ;
#3223=CARTESIAN_POINT ( 'NONE',  ( -10.31217782649100556, 10.00000000000000355, -6.531088913245662653 ) ) ;
#3226=DIRECTION ( 'NONE',  ( 0.000000000000000000, 0.000000000000000000, 1.000000000000000000 ) ) ;
#3229=LINE ( 'NONE', #773, #1544 ) ;
#3236=ORIENTED_EDGE ( 'NONE', *, *, #6458, .F. ) ;
#3239=DIRECTION ( 'NONE',  ( -0.2499999999999979738, 0.8660254037844380415, -0.4330127018922216853 ) ) ;
#3241=FACE_OUTER_BOUND ( 'NONE', #1800, .T. ) ;
#3245=ORIENTED_EDGE ( 'NONE', *, *, #4138, .T. ) ;
#3252=FACE_BOUND ( 'NONE', #6459, .T. ) ;
#3261=ORIENTED_EDGE ( 'NONE', *, *, #5039, .T. ) ;
#3265=ADVANCED_FACE ( 'NONE', ( #4604 ), #9665, .T. ) ;
#3267=CARTESIAN_POINT ( 'NONE',  ( -6.531088913245624461, 10.00000000000000355, 10.31217782649102332 ) ) ;
#3277=DIRECTION ( 'NONE',  ( 0.000000000000000000, 1.000000000000000000, 0.000000000000000000 ) ) ;
#3281=CARTESIAN_POINT ( 'NONE',  ( -6.982120021884462346, 10.00000000000000355, -0.5000000000000731637 ) ) ;
#3288=ORIENTED_EDGE ( 'NONE', *, *, #7488, .F. ) ;
#3296=( NAMED_UNIT ( * ) PLANE_ANGLE_UNIT ( ) SI_UNIT ( $, .RADIAN. ) );
#3298=CARTESIAN_POINT ( 'NONE',  ( -6.982120021884474781, 10.00000000000000355, 0.4999999999999269473 ) ) ;
#3304=VERTEX_POINT ( 'NONE', #2749 ) ;
#3308=VECTOR ( 'NONE', #2819, 1000.000000000000000 ) ;
#3309=ORIENTED_EDGE ( 'NONE', *, *, #7016, .F. ) ;
#3315=ORIENTED_EDGE ( 'NONE', *, *, #5786, .T. ) ;
#3324=DIRECTION ( 'NONE',  ( 0.000000000000000000, 0.000000000000000000, 1.000000000000000000 ) ) ;
#3325=DIRECTION ( 'NONE',  ( 0.000000000000000000, 0.000000000000000000, -1.000000000000000000 ) ) ;
#3328=CARTESIAN_POINT ( 'NONE',  ( -12.19615242270663913, 10.00000000000000355, -0.5000000000001277867 ) ) ;
#3329=CIRCLE ( 'NONE', #7580, 2.149999999999999911 ) ;
#3332=ORIENTED_EDGE ( 'NONE', *, *, #10506, .T. ) ;
#3335=CARTESIAN_POINT ( 'NONE',  ( 13.47724133595216500, 7.781088913245554295, -0.4999999999999529821 ) ) ;
#3338=( BOUNDED_CURVE ( )  B_SPLINE_CURVE ( 3, ( #1563, #2338, #8409, #10911 ),
 .UNSPECIFIED., .F., .F. ) 
 B_SPLINE_CURVE_WITH_KNOTS ( ( 4, 4 ),
 ( 2.284520705739656155, 2.356010155625177127 ),
 .UNSPECIFIED. ) 
 CURVE ( )  GEOMETRIC_REPRESENTATION_ITEM ( )  RATIONAL_B_SPLINE_CURVE ( ( 1.000000000000000000, 0.9995741502243209453, 0.9995741502243209453, 1.000000000000000000 ) ) 
 REPRESENTATION_ITEM ( '' )  );
#3343=FACE_OUTER_BOUND ( 'NONE', #1792, .T. ) ;
#3346=EDGE_LOOP ( 'NONE', ( #5619, #6354, #8668 ) ) ;
#3348=EDGE_CURVE ( 'NONE', #4862, #9084, #701, .T. ) ;
#3358=DIRECTION ( 'NONE',  ( -0.000000000000000000, 1.000000000000000000, -0.000000000000000000 ) ) ;
#3374=PLANE ( 'NONE',  #5190 ) ;
#3389=DIRECTION ( 'NONE',  ( 0.1767766952966340899, 0.3535533905932753407, 0.9185586535436918165 ) ) ;
#3396=CARTESIAN_POINT ( 'NONE',  ( 3.933012701892183660, 10.00000000000000355, 5.812177826491091714 ) ) ;
#3401=EDGE_LOOP ( 'NONE', ( #3024, #1755, #1813, #7534, #1740, #9802 ) ) ;
#3404=EDGE_CURVE ( 'NONE', #915, #20, #10035, .T. ) ;
#3413=CARTESIAN_POINT ( 'NONE',  ( 6.982120021884469452, 19.03096903053430466, -0.4999999999999756306 ) ) ;
#3422=EDGE_CURVE ( 'NONE', #6438, #6764, #7551, .T. ) ;
#3423=EDGE_LOOP ( 'NONE', ( #294, #438, #1799, #4005, #2966, #501 ) ) ;
#3431=DIRECTION ( 'NONE',  ( 0.000000000000000000, 0.000000000000000000, 1.000000000000000000 ) ) ;
#3435=EDGE_CURVE ( 'NONE', #10325, #6438, #992, .T. ) ;
#3444=ORIENTED_EDGE ( 'NONE', *, *, #2281, .T. ) ;
#3449=CARTESIAN_POINT ( 'NONE',  ( 11.42163336986827815, 7.781088913245564953, 7.171633369868360752 ) ) ;
#3452=ORIENTED_EDGE ( 'NONE', *, *, #7252, .T. ) ;
#3454=DIRECTION ( 'NONE',  ( 0.5000000000000009992, -0.8660254037844380415, 1.745740669421570228E-15 ) ) ;
#3459=LINE ( 'NONE', #3281, #3948 ) ;
#3460=FACE_OUTER_BOUND ( 'NONE', #1167, .T. ) ;
#3461=LINE ( 'NONE', #10102, #3109 ) ;
#3462=MECHANICAL_DESIGN_GEOMETRIC_PRESENTATION_REPRESENTATION('',(#9483),#7711);
#3475=CARTESIAN_POINT ( 'NONE',  ( 6.305607966083884186, 7.781088913245563177, -11.92163336986830480 ) ) ;
#3479=VECTOR ( 'NONE', #8259, 1000.000000000000000 ) ;
#3481=EDGE_CURVE ( 'NONE', #7721, #9883, #9878, .T. ) ;
#3483=ORIENTED_EDGE ( 'NONE', *, *, #5251, .F. ) ;
#3492=ORIENTED_EDGE ( 'NONE', *, *, #1270, .T. ) ;
#3495=CARTESIAN_POINT ( 'NONE',  ( -0.5000000000000000000, 0.000000000000000000, 0.000000000000000000 ) ) ;
#3496=CARTESIAN_POINT ( 'NONE',  ( 0.000000000000000000, 7.000000000000003553, 0.000000000000000000 ) ) ;
#3499=DIRECTION ( 'NONE',  ( 0.1889822365046257002, -0.000000000000000000, -0.9819805060619632986 ) ) ;
#3511=PLANE ( 'NONE',  #566 ) ;
#3514=PRODUCT_DEFINITION_FORMATION_WITH_SPECIFIED_SOURCE ( 'ANY', '', #4613, .NOT_KNOWN. ) ;
#3519=CARTESIAN_POINT ( 'NONE',  ( -6.145599950363554775, 19.66631150450992038, -3.355508642977555578 ) ) ;
#3520=CARTESIAN_POINT ( 'NONE',  ( -11.06217782649100734, 10.00000000000000355, -6.386751345948264103 ) ) ;
#3523=CARTESIAN_POINT ( 'NONE',  ( 5.796693311223918066, 19.03096903053432598, -3.924072712834439702 ) ) ;
#3537=DIRECTION ( 'NONE',  ( 0.000000000000000000, 1.000000000000000000, 0.000000000000000000 ) ) ;
#3538=VECTOR ( 'NONE', #1185, 1000.000000000000114 ) ;
#3553=DIRECTION ( 'NONE',  ( 0.000000000000000000, 1.000000000000000000, 0.000000000000000000 ) ) ;
#3559=EDGE_LOOP ( 'NONE', ( #6413, #7496, #8083 ) ) ;
#3560=EDGE_LOOP ( 'NONE', ( #8976, #5605, #7607, #4686 ) ) ;
#3567=CARTESIAN_POINT ( 'NONE',  ( -6.386751345948222358, 10.00000000000000355, 11.06217782649103221 ) ) ;
#3568=AXIS2_PLACEMENT_3D ( 'NONE', #2036, #1984, #3628 ) ;
#3570=LINE ( 'NONE', #8718, #7591 ) ;
#3574=EDGE_LOOP ( 'NONE', ( #9908, #2349, #8533, #9673, #2490, #5984 ) ) ;
#3589=CARTESIAN_POINT ( 'NONE',  ( 0.000000000000000000, 20.00000000000000355, 0.000000000000000000 ) ) ;
#3594=EDGE_LOOP ( 'NONE', ( #4590, #6969, #6282, #8093 ) ) ;
#3597=LINE ( 'NONE', #8622, #8326 ) ;
#3610=PLANE ( 'NONE',  #5678 ) ;
#3611=DIRECTION ( 'NONE',  ( -0.000000000000000000, 1.000000000000000000, -0.000000000000000000 ) ) ;
#3620=ADVANCED_FACE ( 'NONE', ( #8602 ), #7786, .F. ) ;
#3628=DIRECTION ( 'NONE',  ( -0.8660254037844328234, 0.000000000000000000, -0.5000000000000101030 ) ) ;
#3630=ORIENTED_EDGE ( 'NONE', *, *, #2138, .F. ) ;
#3632=EDGE_CURVE ( 'NONE', #3304, #5761, #6709, .T. ) ;
#3633=ORIENTED_EDGE ( 'NONE', *, *, #4017, .F. ) ;
#3636=DIRECTION ( 'NONE',  ( -3.491481338843133355E-15, 0.000000000000000000, 1.000000000000000000 ) ) ;
#3639=LINE ( 'NONE', #5311, #4956 ) ;
#3642=CARTESIAN_POINT ( 'NONE',  ( 0.000000000000000000, 10.00000000000000355, 0.000000000000000000 ) ) ;
#3644=DIRECTION ( 'NONE',  ( 0.000000000000000000, 1.000000000000000000, 0.000000000000000000 ) ) ;
#3649=ORIENTED_EDGE ( 'NONE', *, *, #1464, .F. ) ;
#3650=CARTESIAN_POINT ( 'NONE',  ( -0.2499999999999960032, 0.000000000000000000, -0.4330127018922216298 ) ) ;
#3656=ORIENTED_EDGE ( 'NONE', *, *, #8257, .T. ) ;
#3666=CARTESIAN_POINT ( 'NONE',  ( 3.058047309050022200, 19.03096903053434019, -6.296693311223905631 ) ) ;
#3667=FACE_OUTER_BOUND ( 'NONE', #3156, .T. ) ;
#3677=FACE_OUTER_BOUND ( 'NONE', #6607, .T. ) ;
#3683=DIRECTION ( 'NONE',  ( 0.000000000000000000, -0.000000000000000000, 1.000000000000000000 ) ) ;
#3686=CARTESIAN_POINT ( 'NONE',  ( -10.31217782649113524, 10.00000000000000355, 6.531088913245442384 ) ) ;
#3687=PLANE ( 'NONE',  #5319 ) ;
#3695=FACE_OUTER_BOUND ( 'NONE', #7178, .T. ) ;
#3696=EDGE_CURVE ( 'NONE', #5553, #2787, #8816, .T. ) ;
#3698=ORIENTED_EDGE ( 'NONE', *, *, #3003, .T. ) ;
#3710=CARTESIAN_POINT ( 'NONE',  ( 0.000000000000000000, 7.000000000000003553, 0.000000000000000000 ) ) ;
#3712=CARTESIAN_POINT ( 'NONE',  ( 11.12916512459886675, 10.00000000000000355, -6.580127018922165227 ) ) ;
#3717=VERTEX_POINT ( 'NONE', #9884 ) ;
#3720=LINE ( 'NONE', #8746, #3538 ) ;
#3729=LINE ( 'NONE', #5290, #4242 ) ;
#3730=ORIENTED_EDGE ( 'NONE', *, *, #1584, .T. ) ;
#3736=DIRECTION ( 'NONE',  ( 0.000000000000000000, 0.000000000000000000, 1.000000000000000000 ) ) ;
#3737=CARTESIAN_POINT ( 'NONE',  ( -3.208128317448845301, 19.34316356887878641, -6.223805082245781328 ) ) ;
#3741=AXIS2_PLACEMENT_3D ( 'NONE', #7606, #3277, #10932 ) ;
#3746=CARTESIAN_POINT ( 'NONE',  ( -3.924072712834500543, 10.00000000000000355, 5.796693311223878098 ) ) ;
#3747=LINE ( 'NONE', #7127, #5379 ) ;
#3749=DIRECTION ( 'NONE',  ( 0.000000000000000000, 0.000000000000000000, 1.000000000000000000 ) ) ;
#3753=ORIENTED_EDGE ( 'NONE', *, *, #1741, .F. ) ;
#3770=EDGE_CURVE ( 'NONE', #20, #10157, #5750, .T. ) ;
#3773=ORIENTED_EDGE ( 'NONE', *, *, #8689, .F. ) ;
#3776=EDGE_CURVE ( 'NONE', #10524, #3818, #613, .T. ) ;
#3787=EDGE_CURVE ( 'NONE', #7897, #399, #6690, .T. ) ;
#3789=EDGE_LOOP ( 'NONE', ( #213, #1539, #4820, #4514, #8721, #7694 ) ) ;
#3791=ORIENTED_EDGE ( 'NONE', *, *, #3404, .T. ) ;
#3794=CARTESIAN_POINT ( 'NONE',  ( 1.564302918553086774E-15, 7.000000000000003553, -12.77350269189627063 ) ) ;
#3795=DIRECTION ( 'NONE',  ( -0.000000000000000000, 0.000000000000000000, -1.000000000000000000 ) ) ;
#3797=ORIENTED_EDGE ( 'NONE', *, *, #7898, .F. ) ;
#3799=CARTESIAN_POINT ( 'NONE',  ( -5.237222008264700033E-15, 0.000000000000000000, 0.5000000000000000000 ) ) ;
#3804=CARTESIAN_POINT ( 'NONE',  ( 0.000000000000000000, 10.00000000000000355, 0.000000000000000000 ) ) ;
#3805=ORIENTED_EDGE ( 'NONE', *, *, #1008, .T. ) ;
#3806=ORIENTED_EDGE ( 'NONE', *, *, #9634, .T. ) ;
#3814=ORIENTED_EDGE ( 'NONE', *, *, #4017, .T. ) ;
#3818=VERTEX_POINT ( 'NONE', #2266 ) ;
#3824=CARTESIAN_POINT ( 'NONE',  ( -0.5000000000000000000, 19.03096903053430822, -6.982120021884467675 ) ) ;
#3830=FACE_OUTER_BOUND ( 'NONE', #9551, .T. ) ;
#3840=PRESENTATION_STYLE_ASSIGNMENT (( #4735 ) ) ;
#3845=EDGE_LOOP ( 'NONE', ( #4045, #8485, #8647, #9852, #842, #967 ) ) ;
#3852=DIRECTION ( 'NONE',  ( 0.4999999999999949485, 0.000000000000000000, 0.8660254037844415942 ) ) ;
#3854=CARTESIAN_POINT ( 'NONE',  ( 0.5000000000000000000, 19.03096903053429756, -6.982120021884467675 ) ) ;
#3859=ORIENTED_EDGE ( 'NONE', *, *, #10780, .F. ) ;
#3862=FACE_OUTER_BOUND ( 'NONE', #1378, .T. ) ;
#3864=VERTEX_POINT ( 'NONE', #5976 ) ;
#3873=LINE ( 'NONE', #9681, #3308 ) ;
#3876=ORIENTED_EDGE ( 'NONE', *, *, #3963, .F. ) ;
#3879=CARTESIAN_POINT ( 'NONE',  ( -6.982120021884462346, 19.03096903053432243, -0.5000000000000731637 ) ) ;
#3886=ORIENTED_EDGE ( 'NONE', *, *, #4529, .T. ) ;
#3901=CARTESIAN_POINT ( 'NONE',  ( -3.499999999999921840, 20.00000000000000355, -6.062177826491114807 ) ) ;
#3906=ORIENTED_EDGE ( 'NONE', *, *, #7269, .T. ) ;
#3909=EDGE_CURVE ( 'NONE', #7721, #10062, #7683, .T. ) ;
#3915=DIRECTION ( 'NONE',  ( 0.5000000000000009992, 0.000000000000000000, -0.8660254037844380415 ) ) ;
#3935=VECTOR ( 'NONE', #5261, 1000.000000000000114 ) ;
#3938=VECTOR ( 'NONE', #9906, 1000.000000000000114 ) ;
#3943=FACE_OUTER_BOUND ( 'NONE', #428, .T. ) ;
#3944=DIRECTION ( 'NONE',  ( -0.2499999999999949762, -0.8660254037844380415, -0.4330127018922234061 ) ) ;
#3948=VECTOR ( 'NONE', #1763, 1000.000000000000000 ) ;
#3949=ORIENTED_EDGE ( 'NONE', *, *, #2395, .F. ) ;
#3963=EDGE_CURVE ( 'NONE', #7572, #5862, #4556, .T. ) ;
#3966=EDGE_LOOP ( 'NONE', ( #2040, #6861, #909 ) ) ;
#3967=EDGE_CURVE ( 'NONE', #9358, #8587, #6261, .T. ) ;
#3968=DIRECTION ( 'NONE',  ( 1.047444401652940007E-14, 0.000000000000000000, -1.000000000000000000 ) ) ;
#3972=FACE_OUTER_BOUND ( 'NONE', #2902, .T. ) ;
#3976=ADVANCED_FACE ( 'NONE', ( #10448 ), #3016, .T. ) ;
#3985=DIRECTION ( 'NONE',  ( 0.000000000000000000, 1.000000000000000000, 0.000000000000000000 ) ) ;
#3988=ORIENTED_EDGE ( 'NONE', *, *, #5849, .F. ) ;
#3998=PLANE ( 'NONE',  #2467 ) ;
#4004=CARTESIAN_POINT ( 'NONE',  ( 3.644491357022480837, 19.66631150450990617, 5.978755702618567369 ) ) ;
#4005=ORIENTED_EDGE ( 'NONE', *, *, #1213, .T. ) ;
#4007=DIRECTION ( 'NONE',  ( 0.000000000000000000, 0.000000000000000000, -1.000000000000000000 ) ) ;
#4010=( BOUNDED_CURVE ( )  B_SPLINE_CURVE ( 3, ( #863, #5124, #7714, #9246 ),
 .UNSPECIFIED., .F., .F. ) 
 B_SPLINE_CURVE_WITH_KNOTS ( ( 4, 4 ),
 ( 3.927175151554409549, 3.998664601439929189 ),
 .UNSPECIFIED. ) 
 CURVE ( )  GEOMETRIC_REPRESENTATION_ITEM ( )  RATIONAL_B_SPLINE_CURVE ( ( 1.000000000000000000, 0.9995741502243209453, 0.9995741502243209453, 1.000000000000000000 ) ) 
 REPRESENTATION_ITEM ( '' )  );
#4017=EDGE_CURVE ( 'NONE', #10229, #6293, #9564, .T. ) ;
#4019=EDGE_CURVE ( 'NONE', #7282, #7845, #526, .T. ) ;
#4031=FACE_OUTER_BOUND ( 'NONE', #219, .T. ) ;
#4040=ORIENTED_EDGE ( 'NONE', *, *, #688, .F. ) ;
#4041=VERTEX_POINT ( 'NONE', #6418 ) ;
#4045=ORIENTED_EDGE ( 'NONE', *, *, #9634, .F. ) ;
#4047=CARTESIAN_POINT ( 'NONE',  ( -6.296693311223937606, 19.03096903053434019, 3.058047309049956031 ) ) ;
#4050=LINE ( 'NONE', #1553, #5469 ) ;
#4052=ORIENTED_EDGE ( 'NONE', *, *, #9364, .F. ) ;
#4054=ORIENTED_EDGE ( 'NONE', *, *, #7488, .T. ) ;
#4058=AXIS2_PLACEMENT_3D ( 'NONE', #2823, #5486, #8850 ) ;
#4060=ORIENTED_EDGE ( 'NONE', *, *, #4211, .F. ) ;
#4076=( BOUNDED_CURVE ( )  B_SPLINE_CURVE ( 3, ( #403, #8023, #7149, #3824 ),
 .UNSPECIFIED., .F., .F. ) 
 B_SPLINE_CURVE_WITH_KNOTS ( ( 4, 4 ),
 ( 2.284520705739656155, 2.356010155625177127 ),
 .UNSPECIFIED. ) 
 CURVE ( )  GEOMETRIC_REPRESENTATION_ITEM ( )  RATIONAL_B_SPLINE_CURVE ( ( 1.000000000000000000, 0.9995741502243209453, 0.9995741502243209453, 1.000000000000000000 ) ) 
 REPRESENTATION_ITEM ( '' )  );
#4079=VERTEX_POINT ( 'NONE', #1327 ) ;
#4080=DIRECTION ( 'NONE',  ( 0.2500000000000041078, 0.8660254037844380415, -0.4330127018922182436 ) ) ;
#4084=ORIENTED_EDGE ( 'NONE', *, *, #8149, .T. ) ;
#4086=LINE ( 'NONE', #10764, #54 ) ;
#4088=FACE_OUTER_BOUND ( 'NONE', #10572, .T. ) ;
#4094=ADVANCED_FACE ( 'NONE', ( #4508 ), #287, .T. ) ;
#4105=CARTESIAN_POINT ( 'NONE',  ( 0.000000000000000000, 10.00000000000000355, 0.000000000000000000 ) ) ;
#4106=CARTESIAN_POINT ( 'NONE',  ( -3.924072712834500543, 19.03096903053431177, 5.796693311223878098 ) ) ;
#4107=DIRECTION ( 'NONE',  ( 0.000000000000000000, 0.000000000000000000, 1.000000000000000000 ) ) ;
#4121=CARTESIAN_POINT ( 'NONE',  ( 0.000000000000000000, 10.00000000000000355, 0.000000000000000000 ) ) ;
#4123=CARTESIAN_POINT ( 'NONE',  ( 2.632990618166809235E-16, 20.00000000000000355, 2.149999999999999911 ) ) ;
#4129=AXIS2_PLACEMENT_3D ( 'NONE', #8373, #4295, #1747 ) ;
#4137=ORIENTED_EDGE ( 'NONE', *, *, #453, .T. ) ;
#4138=EDGE_CURVE ( 'NONE', #528, #2606, #604, .T. ) ;
#4139=LINE ( 'NONE', #4358, #5627 ) ;
#4143=ORIENTED_EDGE ( 'NONE', *, *, #4218, .T. ) ;
#4144=DIRECTION ( 'NONE',  ( 0.000000000000000000, 0.000000000000000000, -1.000000000000000000 ) ) ;
#4146=DIRECTION ( 'NONE',  ( 0.2499999999999979738, -0.8660254037844380415, 0.4330127018922216853 ) ) ;
#4163=EDGE_CURVE ( 'NONE', #689, #10532, #768, .T. ) ;
#4166=CARTESIAN_POINT ( 'NONE',  ( 6.982120021884469452, 10.00000000000000355, -0.4999999999999756306 ) ) ;
#4177=CARTESIAN_POINT ( 'NONE',  ( -0.5000000000000000000, 10.00000000000000355, 5.999999999999998224 ) ) ;
#4179=FACE_OUTER_BOUND ( 'NONE', #660, .T. ) ;
#4184=CARTESIAN_POINT ( 'NONE',  ( 0.000000000000000000, 10.00000000000000355, 0.000000000000000000 ) ) ;
#4185=DIRECTION ( 'NONE',  ( 0.000000000000000000, -1.000000000000000000, 0.000000000000000000 ) ) ;
#4186=CARTESIAN_POINT ( 'NONE',  ( 3.924072712834419718, 19.03096903053430466, 5.796693311223933165 ) ) ;
#4187=DIRECTION ( 'NONE',  ( 0.2499999999999949762, 0.8660254037844380415, 0.4330127018922234061 ) ) ;
#4193=FACE_OUTER_BOUND ( 'NONE', #3423, .T. ) ;
#4195=VECTOR ( 'NONE', #8534, 1000.000000000000000 ) ;
#4211=EDGE_CURVE ( 'NONE', #5713, #2855, #7948, .T. ) ;
#4218=EDGE_CURVE ( 'NONE', #7303, #10062, #3329, .T. ) ;
#4223=ORIENTED_EDGE ( 'NONE', *, *, #6731, .F. ) ;
#4224=ORIENTED_EDGE ( 'NONE', *, *, #1199, .T. ) ;
#4225=ORIENTED_EDGE ( 'NONE', *, *, #7734, .T. ) ;
#4240=ADVANCED_FACE ( 'NONE', ( #4031 ), #2248, .F. ) ;
#4242=VECTOR ( 'NONE', #3611, 1000.000000000000000 ) ;
#4243=DIRECTION ( 'NONE',  ( 0.4999999999999949485, 0.000000000000000000, 0.8660254037844415942 ) ) ;
#4248=CARTESIAN_POINT ( 'NONE',  ( 0.000000000000000000, 10.00000000000000355, 0.000000000000000000 ) ) ;
#4267=ORIENTED_EDGE ( 'NONE', *, *, #4582, .T. ) ;
#4278=DIRECTION ( 'NONE',  ( 0.000000000000000000, 1.000000000000000000, 0.000000000000000000 ) ) ;
#4284=AXIS2_PLACEMENT_3D ( 'NONE', #6177, #7715, #3736 ) ;
#4285=ORIENTED_EDGE ( 'NONE', *, *, #8359, .F. ) ;
#4287=ORIENTED_EDGE ( 'NONE', *, *, #8335, .F. ) ;
#4292=CARTESIAN_POINT ( 'NONE',  ( 1.745740669421566678E-15, 0.000000000000000000, -0.5000000000000000000 ) ) ;
#4295=DIRECTION ( 'NONE',  ( 0.000000000000000000, 1.000000000000000000, 0.000000000000000000 ) ) ;
#4300=COLOUR_RGB ( '', 0.40784314, 0.44705882, 0.49803922) ;
#4306=CARTESIAN_POINT ( 'NONE',  ( 6.999999999999999112, 10.00000000000000355, -0.4999999999999756306 ) ) ;
#4353=PLANE ( 'NONE',  #34 ) ;
#4355=EDGE_LOOP ( 'NONE', ( #3026, #6096, #2981 ) ) ;
#4358=CARTESIAN_POINT ( 'NONE',  ( 3.058047309050022200, 10.00000000000000355, -6.296693311223905631 ) ) ;
#4361=ORIENTED_EDGE ( 'NONE', *, *, #3348, .T. ) ;
#4362=FACE_OUTER_BOUND ( 'NONE', #3845, .T. ) ;
#4365=FACE_OUTER_BOUND ( 'NONE', #9338, .T. ) ;
#4376=EDGE_LOOP ( 'NONE', ( #1409, #4874, #4740, #6629 ) ) ;
#4380=CLOSED_SHELL ( 'NONE', ( #5819, #4792, #7310, #5451, #5645, #6966, #5540, #6066, #5508, #4402, #8300, #144, #2259, #1666, #3976, #8140, #5729, #5339, #1872, #2330, #8019, #5863, #9753, #628, #8569, #1883, #6678, #7600, #3265, #10809, #1826, #9898, #9827, #9437, #1802, #9909, #2814, #8162, #10752, #6732, #2059, #8709, #8758, #6536, #8613, #3620, #8464, #2737, #4094, #4527, #2726, #6521, #2586, #9633, #10442, #8085, #5657, #2759, #5921, #1001, #9597, #4240, #9450, #9497, #5446, #818, #10376, #9637, #4541, #10262, #643, #5445, #9047, #7871, #6683, #2603, #8819, #6464, #1570, #3111, #309 ) ) ;
#4388=VECTOR ( 'NONE', #2926, 1000.000000000000000 ) ;
#4389=CARTESIAN_POINT ( 'NONE',  ( -7.171633369868158248, 7.781088913245561400, -11.42163336986839717 ) ) ;
#4396=EDGE_CURVE ( 'NONE', #417, #915, #8518, .T. ) ;
#4398=FACE_OUTER_BOUND ( 'NONE', #9766, .T. ) ;
#4402=ADVANCED_FACE ( 'NONE', ( #4362 ), #7608, .T. ) ;
#4410=EDGE_CURVE ( 'NONE', #3051, #10524, #41, .T. ) ;
#4425=DIRECTION ( 'NONE',  ( 0.000000000000000000, -0.000000000000000000, 1.000000000000000000 ) ) ;
#4429=AXIS2_PLACEMENT_3D ( 'NONE', #4105, #3136, #6591 ) ;
#4433=VECTOR ( 'NONE', #6115, 1000.000000000000000 ) ;
#4439=VERTEX_POINT ( 'NONE', #5032 ) ;
#4459=ORIENTED_EDGE ( 'NONE', *, *, #6483, .T. ) ;
#4462=DIRECTION ( 'NONE',  ( 0.000000000000000000, 0.000000000000000000, 1.000000000000000000 ) ) ;
#4468=VERTEX_POINT ( 'NONE', #1934 ) ;
#4471=ORIENTED_EDGE ( 'NONE', *, *, #446, .F. ) ;
#4474=AXIS2_PLACEMENT_3D ( 'NONE', #3799, #3968, #588 ) ;
#4493=VECTOR ( 'NONE', #7965, 1000.000000000000000 ) ;
#4498=CARTESIAN_POINT ( 'NONE',  ( 5.510910596163089556E-16, 7.000000000000003553, 4.500000000000000888 ) ) ;
#4500=ORIENTED_EDGE ( 'NONE', *, *, #45, .T. ) ;
#4508=FACE_OUTER_BOUND ( 'NONE', #10136, .T. ) ;
#4514=ORIENTED_EDGE ( 'NONE', *, *, #1516, .T. ) ;
#4515=ORIENTED_EDGE ( 'NONE', *, *, #9702, .T. ) ;
#4527=ADVANCED_FACE ( 'NONE', ( #7852 ), #1263, .F. ) ;
#4529=EDGE_CURVE ( 'NONE', #10532, #2855, #3639, .T. ) ;
#4531=EDGE_LOOP ( 'NONE', ( #2723, #2908, #429, #8303 ) ) ;
#4532=LINE ( 'NONE', #9298, #9122 ) ;
#4541=ADVANCED_FACE ( 'NONE', ( #4547 ), #2849, .T. ) ;
#4542=FACE_OUTER_BOUND ( 'NONE', #4355, .T. ) ;
#4547=FACE_OUTER_BOUND ( 'NONE', #2930, .T. ) ;
#4551=ORIENTED_EDGE ( 'NONE', *, *, #1680, .F. ) ;
#4552=CARTESIAN_POINT ( 'NONE',  ( 0.000000000000000000, 10.10000000000000497, 0.000000000000000000 ) ) ;
#4554=CARTESIAN_POINT ( 'NONE',  ( 6.145599950363579644, 19.66631150450992038, 3.355508642977511613 ) ) ;
#4555=EDGE_LOOP ( 'NONE', ( #9093, #524, #2548 ) ) ;
#4556=LINE ( 'NONE', #5473, #5119 ) ;
#4561=VERTEX_POINT ( 'NONE', #3746 ) ;
#4565=CARTESIAN_POINT ( 'NONE',  ( 10.81217782649109083, 10.00000000000000355, -5.665063509461074176 ) ) ;
#4573=CARTESIAN_POINT ( 'NONE',  ( 6.223805082245746689, 19.34316356887877930, -3.208128317448911915 ) ) ;
#4574=DIRECTION ( 'NONE',  ( 0.8660254037844363761, 0.000000000000000000, 0.5000000000000039968 ) ) ;
#4577=VECTOR ( 'NONE', #8672, 1000.000000000000000 ) ;
#4582=EDGE_CURVE ( 'NONE', #9521, #9309, #9556, .T. ) ;
#4586=CARTESIAN_POINT ( 'NONE',  ( -5.796693311223863887, 19.03096903053432598, -3.924072712834521415 ) ) ;
#4588=DIRECTION ( 'NONE',  ( 0.5000000000000009992, -0.8660254037844380415, 1.745740669421570228E-15 ) ) ;
#4590=ORIENTED_EDGE ( 'NONE', *, *, #9702, .F. ) ;
#4592=AXIS2_PLACEMENT_3D ( 'NONE', #7635, #244, #903 ) ;
#4604=FACE_OUTER_BOUND ( 'NONE', #3789, .T. ) ;
#4605=FACE_OUTER_BOUND ( 'NONE', #8470, .T. ) ;
#4612=CARTESIAN_POINT ( 'NONE',  ( 5.796693311223918954, 10.00000000000000355, -3.924072712834440591 ) ) ;
#4613=PRODUCT ( 'Inner Conical Burr Core', 'Inner Conical Burr Core', '', ( #8213 ) ) ;
#4617=DIRECTION ( 'NONE',  ( 0.000000000000000000, 0.000000000000000000, 1.000000000000000000 ) ) ;
#4622=LINE ( 'NONE', #10517, #4388 ) ;
#4623=PLANE ( 'NONE',  #5314 ) ;
#4628=VERTEX_POINT ( 'NONE', #1112 ) ;
#4631=DIRECTION ( 'NONE',  ( 0.000000000000000000, 1.000000000000000000, 0.000000000000000000 ) ) ;
#4634=LINE ( 'NONE', #7989, #1104 ) ;
#4635=CARTESIAN_POINT ( 'NONE',  ( 0.4330127018922190207, 0.000000000000000000, 0.2500000000000004996 ) ) ;
#4643=PLANE ( 'NONE',  #7981 ) ;
#4653=ORIENTED_EDGE ( 'NONE', *, *, #6507, .T. ) ;
#4655=AXIS2_PLACEMENT_3D ( 'NONE', #2692, #6025, #5085 ) ;
#4657=CARTESIAN_POINT ( 'NONE',  ( 3.058047309050022200, 19.03096903053434019, -6.296693311223905631 ) ) ;
#4666=LINE ( 'NONE', #3712, #5620 ) ;
#4667=ORIENTED_EDGE ( 'NONE', *, *, #396, .F. ) ;
#4682=EDGE_CURVE ( 'NONE', #1319, #375, #6556, .T. ) ;
#4684=ORIENTED_EDGE ( 'NONE', *, *, #525, .T. ) ;
#4685=ORIENTED_EDGE ( 'NONE', *, *, #9364, .T. ) ;
#4686=ORIENTED_EDGE ( 'NONE', *, *, #5257, .T. ) ;
#4691=CARTESIAN_POINT ( 'NONE',  ( 6.062177826491051746, 20.00000000000000355, 3.500000000000027089 ) ) ;
#4694=EDGE_LOOP ( 'NONE', ( #200, #1493, #8368 ) ) ;
#4696=EDGE_LOOP ( 'NONE', ( #6553, #1074, #732 ) ) ;
#4700=CARTESIAN_POINT ( 'NONE',  ( -3.058047309049933382, 19.03096903053431532, -6.296693311223948264 ) ) ;
#4702=EDGE_CURVE ( 'NONE', #1515, #7572, #10589, .T. ) ;
#4715=EDGE_LOOP ( 'NONE', ( #4285, #4868 ) ) ;
#4724=DIRECTION ( 'NONE',  ( 0.4999999999999949485, 0.000000000000000000, 0.8660254037844415942 ) ) ;
#4725=CARTESIAN_POINT ( 'NONE',  ( 5.937177826491071286, 19.75000000000000000, -2.850480947161653233 ) ) ;
#4733=EDGE_CURVE ( 'NONE', #9084, #620, #9775, .T. ) ;
#4735=SURFACE_STYLE_USAGE ( .BOTH. , #6638 ) ;
#4737=DIRECTION ( 'NONE',  ( -0.5000000000000069944, 0.000000000000000000, 0.8660254037844344888 ) ) ;
#4738=CARTESIAN_POINT ( 'NONE',  ( 0.000000000000000000, 10.00000000000000355, 0.000000000000000000 ) ) ;
#4739=CARTESIAN_POINT ( 'NONE',  ( -6.982120021884473005, 10.00000000000000355, 0.4999999999999268363 ) ) ;
#4740=ORIENTED_EDGE ( 'NONE', *, *, #7594, .F. ) ;
#4747=DIRECTION ( 'NONE',  ( 0.000000000000000000, -1.000000000000000000, 0.000000000000000000 ) ) ;
#4750=CIRCLE ( 'NONE', #7558, 6.999999999999997335 ) ;
#4751=ORIENTED_EDGE ( 'NONE', *, *, #9507, .T. ) ;
#4753=DIRECTION ( 'NONE',  ( 0.000000000000000000, -0.8660254037844380415, 0.5000000000000009992 ) ) ;
#4758=DIRECTION ( 'NONE',  ( -0.000000000000000000, -0.8660254037844380415, -0.5000000000000009992 ) ) ;
#4762=ORIENTED_EDGE ( 'NONE', *, *, #5039, .F. ) ;
#4770=EDGE_CURVE ( 'NONE', #10229, #5566, #334, .T. ) ;
#4778=ORIENTED_EDGE ( 'NONE', *, *, #1516, .F. ) ;
#4791=CYLINDRICAL_SURFACE ( 'NONE', #6574, 6.999999999999997335 ) ;
#4792=ADVANCED_FACE ( 'NONE', ( #10923 ), #1636, .F. ) ;
#4794=( BOUNDED_CURVE ( )  B_SPLINE_CURVE ( 3, ( #925, #7658, #89, #10197 ),
 .UNSPECIFIED., .F., .F. ) 
 B_SPLINE_CURVE_WITH_KNOTS ( ( 4, 4 ),
 ( 3.927175151554405996, 3.998664601439927413 ),
 .UNSPECIFIED. ) 
 CURVE ( )  GEOMETRIC_REPRESENTATION_ITEM ( )  RATIONAL_B_SPLINE_CURVE ( ( 1.000000000000000000, 0.9995741502243209453, 0.9995741502243209453, 1.000000000000000000 ) ) 
 REPRESENTATION_ITEM ( '' )  );
#4805=ORIENTED_EDGE ( 'NONE', *, *, #7904, .T. ) ;
#4806=ORIENTED_EDGE ( 'NONE', *, *, #307, .F. ) ;
#4812=AXIS2_PLACEMENT_3D ( 'NONE', #7669, #2405, #10150 ) ;
#4813=DIRECTION ( 'NONE',  ( 0.000000000000000000, 0.000000000000000000, -1.000000000000000000 ) ) ;
#4819=EDGE_LOOP ( 'NONE', ( #7719, #3805, #4143, #10656 ) ) ;
#4820=ORIENTED_EDGE ( 'NONE', *, *, #5121, .F. ) ;
#4831=AXIS2_PLACEMENT_3D ( 'NONE', #2936, #4631, #6339 ) ;
#4834=AXIS2_PLACEMENT_3D ( 'NONE', #9043, #7271, #10747 ) ;
#4837=ORIENTED_EDGE ( 'NONE', *, *, #1584, .F. ) ;
#4840=ORIENTED_EDGE ( 'NONE', *, *, #5121, .T. ) ;
#4841=EDGE_CURVE ( 'NONE', #10217, #9174, #4010, .T. ) ;
#4844=VECTOR ( 'NONE', #9431, 1000.000000000000114 ) ;
#4851=ORIENTED_EDGE ( 'NONE', *, *, #6336, .F. ) ;
#4858=DIRECTION ( 'NONE',  ( -0.000000000000000000, -1.000000000000000000, -0.000000000000000000 ) ) ;
#4862=VERTEX_POINT ( 'NONE', #3267 ) ;
#4868=ORIENTED_EDGE ( 'NONE', *, *, #7734, .F. ) ;
#4873=VERTEX_POINT ( 'NONE', #1806 ) ;
#4874=ORIENTED_EDGE ( 'NONE', *, *, #1270, .F. ) ;
#4879=DIRECTION ( 'NONE',  ( 0.4330127018922172444, 0.8660254037844380415, 0.2500000000000055511 ) ) ;
#4880=CARTESIAN_POINT ( 'NONE',  ( -6.296693311223874545, 19.03096903053432598, -3.058047309050087925 ) ) ;
#4889=DIRECTION ( 'NONE',  ( 0.000000000000000000, 1.000000000000000000, 0.000000000000000000 ) ) ;
#4890=DIRECTION ( 'NONE',  ( -0.000000000000000000, 1.000000000000000000, -0.000000000000000000 ) ) ;
#4892=CARTESIAN_POINT ( 'NONE',  ( 0.000000000000000000, 10.00000000000000355, 0.000000000000000000 ) ) ;
#4900=LINE ( 'NONE', #4177, #6409 ) ;
#4906=LINE ( 'NONE', #5626, #2151 ) ;
#4910=ORIENTED_EDGE ( 'NONE', *, *, #5514, .T. ) ;
#4911=VECTOR ( 'NONE', #5061, 1000.000000000000114 ) ;
#4915=CARTESIAN_POINT ( 'NONE',  ( -0.5000000000000000000, 10.00000000000000355, -6.999999999999997335 ) ) ;
#4919=VECTOR ( 'NONE', #1069, 1000.000000000000000 ) ;
#4932=( NAMED_UNIT ( * ) SI_UNIT ( $, .STERADIAN. ) SOLID_ANGLE_UNIT ( ) );
#4936=DIRECTION ( 'NONE',  ( 0.000000000000000000, 0.000000000000000000, 1.000000000000000000 ) ) ;
#4938=CARTESIAN_POINT ( 'NONE',  ( 0.000000000000000000, 10.00000000000000355, 0.000000000000000000 ) ) ;
#4940=ORIENTED_EDGE ( 'NONE', *, *, #4163, .F. ) ;
#4950=FACE_OUTER_BOUND ( 'NONE', #4696, .T. ) ;
#4951=CARTESIAN_POINT ( 'NONE',  ( 6.386751345948063374, 10.00000000000000355, 11.06217782649112458 ) ) ;
#4953=PLANE ( 'NONE',  #8869 ) ;
#4956=VECTOR ( 'NONE', #5370, 1000.000000000000000 ) ;
#4960=CARTESIAN_POINT ( 'NONE',  ( -6.994037468151973691, 19.34316356887879351, 0.3335819196118008922 ) ) ;
#4984=CARTESIAN_POINT ( 'NONE',  ( 6.531088913245477023, 10.00000000000000355, 10.31217782649111214 ) ) ;
#4998=ORIENTED_EDGE ( 'NONE', *, *, #1016, .F. ) ;
#5010=CYLINDRICAL_SURFACE ( 'NONE', #384, 6.999999999999997335 ) ;
#5014=ORIENTED_EDGE ( 'NONE', *, *, #9010, .F. ) ;
#5020=CARTESIAN_POINT ( 'NONE',  ( -3.058047309050066165, 10.00000000000000355, 6.296693311223885203 ) ) ;
#5026=LINE ( 'NONE', #757, #2672 ) ;
#5027=ORIENTED_EDGE ( 'NONE', *, *, #3220, .T. ) ;
#5030=CARTESIAN_POINT ( 'NONE',  ( -3.499999999999921396, 20.00000000000000355, -6.062177826491113919 ) ) ;
#5032=CARTESIAN_POINT ( 'NONE',  ( 0.5000000000000000000, 19.03096903053430822, 6.982120021884467675 ) ) ;
#5035=CARTESIAN_POINT ( 'NONE',  ( 6.305607966083798921, 7.781088913245563177, 11.92163336986834743 ) ) ;
#5039=EDGE_CURVE ( 'NONE', #1319, #9255, #8715, .T. ) ;
#5045=SURFACE_STYLE_USAGE ( .BOTH. , #6752 ) ;
#5048=LINE ( 'NONE', #2324, #9378 ) ;
#5049=DIRECTION ( 'NONE',  ( -0.5000000000000069944, 0.000000000000000000, 0.8660254037844344888 ) ) ;
#5050=EDGE_CURVE ( 'NONE', #2606, #8513, #7836, .T. ) ;
#5061=DIRECTION ( 'NONE',  ( -0.4330127018922172999, -0.8660254037844380415, -0.2500000000000054956 ) ) ;
#5066=DIRECTION ( 'NONE',  ( 0.000000000000000000, -0.8660254037844380415, -0.5000000000000009992 ) ) ;
#5069=ORIENTED_EDGE ( 'NONE', *, *, #1129, .T. ) ;
#5072=CARTESIAN_POINT ( 'NONE',  ( 0.000000000000000000, 7.000000000000003553, 0.000000000000000000 ) ) ;
#5085=DIRECTION ( 'NONE',  ( 0.000000000000000000, 0.000000000000000000, 1.000000000000000000 ) ) ;
#5092=ORIENTED_EDGE ( 'NONE', *, *, #7757, .T. ) ;
#5099=ORIENTED_EDGE ( 'NONE', *, *, #797, .F. ) ;
#5101=VERTEX_POINT ( 'NONE', #626 ) ;
#5112=DIRECTION ( 'NONE',  ( 0.7071067811865470176, 0.3535533905932748411, -0.6123724356957946924 ) ) ;
#5117=ORIENTED_EDGE ( 'NONE', *, *, #8221, .F. ) ;
#5119=VECTOR ( 'NONE', #2863, 1000.000000000000114 ) ;
#5120=CIRCLE ( 'NONE', #4429, 6.999999999999997335 ) ;
#5121=EDGE_CURVE ( 'NONE', #399, #3717, #775, .T. ) ;
#5123=ORIENTED_EDGE ( 'NONE', *, *, #9421, .T. ) ;
#5124=CARTESIAN_POINT ( 'NONE',  ( 3.208128317448888378, 19.34316356887880772, 6.223805082245760012 ) ) ;
#5127=CARTESIAN_POINT ( 'NONE',  ( 5.510910596163089556E-16, 10.10000000000000497, 4.500000000000000888 ) ) ;
#5128=DIRECTION ( 'NONE',  ( 0.9819805060619676285, 0.000000000000000000, -0.1889822365046036623 ) ) ;
#5142=DIRECTION ( 'NONE',  ( 0.000000000000000000, -0.000000000000000000, -1.000000000000000000 ) ) ;
#5143=EDGE_LOOP ( 'NONE', ( #2724, #10053, #1091, #3698 ) ) ;
#5147=VECTOR ( 'NONE', #4879, 1000.000000000000114 ) ;
#5150=DIRECTION ( 'NONE',  ( 0.000000000000000000, -0.000000000000000000, 1.000000000000000000 ) ) ;
#5164=VERTEX_POINT ( 'NONE', #573 ) ;
#5190=AXIS2_PLACEMENT_3D ( 'NONE', #1565, #3207, #6778 ) ;
#5192=VERTEX_POINT ( 'NONE', #3204 ) ;
#5198=VECTOR ( 'NONE', #694, 1000.000000000000000 ) ;
#5217=EDGE_LOOP ( 'NONE', ( #1092, #291, #10693, #5926, #603, #3195, #3236, #7908, #10400 ) ) ;
#5227=EDGE_CURVE ( 'NONE', #7707, #7572, #9205, .T. ) ;
#5234=DIRECTION ( 'NONE',  ( -0.8838834764831809965, 0.3535533905932741749, -0.3061862178479068386 ) ) ;
#5235=CARTESIAN_POINT ( 'NONE',  ( -0.5000000000000000000, 10.00000000000000355, -12.19615242270663735 ) ) ;
#5247=LINE ( 'NONE', #3567, #4844 ) ;
#5249=PLANE ( 'NONE',  #6017 ) ;
#5250=PLANE ( 'NONE',  #3568 ) ;
#5251=EDGE_CURVE ( 'NONE', #7391, #2965, #3597, .T. ) ;
#5256=ORIENTED_EDGE ( 'NONE', *, *, #5786, .F. ) ;
#5257=EDGE_CURVE ( 'NONE', #9174, #5713, #10014, .T. ) ;
#5258=CARTESIAN_POINT ( 'NONE',  ( -6.296693311223874545, 19.03096903053432598, -3.058047309050087925 ) ) ;
#5259=EDGE_CURVE ( 'NONE', #8587, #4079, #9183, .T. ) ;
#5261=DIRECTION ( 'NONE',  ( -0.5000000000000069944, 0.000000000000000000, 0.8660254037844344888 ) ) ;
#5262=EDGE_CURVE ( 'NONE', #9883, #7721, #943, .T. ) ;
#5264=VECTOR ( 'NONE', #9926, 1000.000000000000000 ) ;
#5267=ORIENTED_EDGE ( 'NONE', *, *, #1016, .T. ) ;
#5273=DIRECTION ( 'NONE',  ( 0.000000000000000000, 0.000000000000000000, 1.000000000000000000 ) ) ;
#5275=EDGE_CURVE ( 'NONE', #10413, #1987, #1621, .T. ) ;
#5289=CARTESIAN_POINT ( 'NONE',  ( 6.296693311223917178, 10.00000000000000355, -3.058047309049999996 ) ) ;
#5290=CARTESIAN_POINT ( 'NONE',  ( 0.000000000000000000, 7.000000000000003553, 12.77350269189627063 ) ) ;
#5294=ORIENTED_EDGE ( 'NONE', *, *, #8221, .T. ) ;
#5296=CARTESIAN_POINT ( 'NONE',  ( -3.355508642977535150, 19.66631150450993104, 6.145599950363565434 ) ) ;
#5311=CARTESIAN_POINT ( 'NONE',  ( 9.633606397919612263, 10.00000000000000355, 2.262820851736541350 ) ) ;
#5314=AXIS2_PLACEMENT_3D ( 'NONE', #10677, #2063, #3035 ) ;
#5319=AXIS2_PLACEMENT_3D ( 'NONE', #1870, #988, #7067 ) ;
#5329=CIRCLE ( 'NONE', #8663, 12.77350269189627063 ) ;
#5335=DIRECTION ( 'NONE',  ( 0.6546536707079774198, -0.000000000000000000, 0.7559289460184541731 ) ) ;
#5339=ADVANCED_FACE ( 'NONE', ( #4088 ), #9102, .T. ) ;
#5341=FACE_OUTER_BOUND ( 'NONE', #8462, .T. ) ;
#5344=LINE ( 'NONE', #10357, #7633 ) ;
#5360=DIRECTION ( 'NONE',  ( 0.000000000000000000, 0.8660254037844380415, -0.5000000000000009992 ) ) ;
#5370=DIRECTION ( 'NONE',  ( 0.3273268353539895426, -0.000000000000000000, 0.9449111825230677164 ) ) ;
#5378=DIRECTION ( 'NONE',  ( 0.000000000000000000, -1.000000000000000000, 0.000000000000000000 ) ) ;
#5379=VECTOR ( 'NONE', #10270, 1000.000000000000114 ) ;
#5383=CARTESIAN_POINT ( 'NONE',  ( 0.000000000000000000, 10.00000000000000355, 0.000000000000000000 ) ) ;
#5402=EDGE_LOOP ( 'NONE', ( #1918, #9571, #829, #4685, #7758, #1689 ) ) ;
#5404=EDGE_CURVE ( 'NONE', #7897, #1247, #606, .T. ) ;
#5410=DIRECTION ( 'NONE',  ( 0.000000000000000000, -0.000000000000000000, 1.000000000000000000 ) ) ;
#5412=DIRECTION ( 'NONE',  ( 0.000000000000000000, 0.000000000000000000, 1.000000000000000000 ) ) ;
#5418=PLANE ( 'NONE',  #6410 ) ;
#5422=DIRECTION ( 'NONE',  ( -0.000000000000000000, 1.000000000000000000, -0.000000000000000000 ) ) ;
#5444=ORIENTED_EDGE ( 'NONE', *, *, #10019, .F. ) ;
#5445=ADVANCED_FACE ( 'NONE', ( #7387 ), #5795, .F. ) ;
#5446=ADVANCED_FACE ( 'NONE', ( #772 ), #9933, .T. ) ;
#5449=AXIS2_PLACEMENT_3D ( 'NONE', #1893, #895, #8623 ) ;
#5451=ADVANCED_FACE ( 'NONE', ( #4193 ), #9058, .T. ) ;
#5452=CARTESIAN_POINT ( 'NONE',  ( 5.796693311223892309, 19.03096903053431532, 3.924072712834481447 ) ) ;
#5459=EDGE_CURVE ( 'NONE', #8414, #6293, #5637, .T. ) ;
#5466=VECTOR ( 'NONE', #10604, 1000.000000000000114 ) ;
#5469=VECTOR ( 'NONE', #671, 1000.000000000000000 ) ;
#5471=EDGE_CURVE ( 'NONE', #2423, #3051, #9401, .T. ) ;
#5473=CARTESIAN_POINT ( 'NONE',  ( 0.1339745962155587111, 10.00000000000000355, 12.92820323027550700 ) ) ;
#5477=DIRECTION ( 'NONE',  ( 0.000000000000000000, -1.000000000000000000, 0.000000000000000000 ) ) ;
#5478=AXIS2_PLACEMENT_3D ( 'NONE', #2083, #432, #2898 ) ;
#5486=DIRECTION ( 'NONE',  ( 0.000000000000000000, 1.000000000000000000, 0.000000000000000000 ) ) ;
#5500=CARTESIAN_POINT ( 'NONE',  ( 0.000000000000000000, 7.000000000000003553, 0.000000000000000000 ) ) ;
#5501=EDGE_CURVE ( 'NONE', #9763, #8026, #8436, .T. ) ;
#5502=FACE_OUTER_BOUND ( 'NONE', #1933, .T. ) ;
#5505=ORIENTED_EDGE ( 'NONE', *, *, #10696, .T. ) ;
#5508=ADVANCED_FACE ( 'NONE', ( #4365 ), #6977, .T. ) ;
#5512=DIRECTION ( 'NONE',  ( 0.000000000000000000, 0.000000000000000000, 1.000000000000000000 ) ) ;
#5514=EDGE_CURVE ( 'NONE', #4041, #1319, #9003, .T. ) ;
#5515=DIRECTION ( 'NONE',  ( 0.000000000000000000, 0.8660254037844380415, 0.5000000000000009992 ) ) ;
#5521=STYLED_ITEM ( 'NONE', ( #3840 ), #7050 ) ;
#5525=CARTESIAN_POINT ( 'NONE',  ( -0.5000000000000000000, 7.781088913245554295, 13.47724133595216323 ) ) ;
#5531=ORIENTED_EDGE ( 'NONE', *, *, #1434, .F. ) ;
#5537=EDGE_LOOP ( 'NONE', ( #3649, #819, #6486, #3906, #1245, #1611 ) ) ;
#5538=ORIENTED_EDGE ( 'NONE', *, *, #8141, .F. ) ;
#5540=ADVANCED_FACE ( 'NONE', ( #3460 ), #6919, .T. ) ;
#5551=FACE_OUTER_BOUND ( 'NONE', #7586, .T. ) ;
#5553=VERTEX_POINT ( 'NONE', #9504 ) ;
#5557=CARTESIAN_POINT ( 'NONE',  ( -3.058047309050066165, 19.03096903053433309, 6.296693311223885203 ) ) ;
#5559=CARTESIAN_POINT ( 'NONE',  ( 6.386751345948143310, 10.00000000000000355, -11.06217782649107839 ) ) ;
#5561=CARTESIAN_POINT ( 'NONE',  ( -0.4330127018922172999, 0.000000000000000000, -0.2500000000000036082 ) ) ;
#5562=PLANE ( 'NONE',  #2997 ) ;
#5566=VERTEX_POINT ( 'NONE', #9258 ) ;
#5571=DIRECTION ( 'NONE',  ( 0.9185586535436925937, 0.3535533905932736198, -0.1767766952966332017 ) ) ;
#5583=CARTESIAN_POINT ( 'NONE',  ( 6.994037468151971915, 19.34316356887878641, -0.3335819196118459673 ) ) ;
#5588=ORIENTED_EDGE ( 'NONE', *, *, #26, .T. ) ;
#5592=CARTESIAN_POINT ( 'NONE',  ( -6.580127018922051541, 10.00000000000000355, -11.12916512459894314 ) ) ;
#5598=FACE_OUTER_BOUND ( 'NONE', #4555, .T. ) ;
#5605=ORIENTED_EDGE ( 'NONE', *, *, #7749, .F. ) ;
#5619=ORIENTED_EDGE ( 'NONE', *, *, #8980, .F. ) ;
#5620=VECTOR ( 'NONE', #8018, 1000.000000000000114 ) ;
#5623=FACE_OUTER_BOUND ( 'NONE', #7560, .T. ) ;
#5626=CARTESIAN_POINT ( 'NONE',  ( 5.812177826491076615, 10.00000000000000355, -3.933012701892204532 ) ) ;
#5627=VECTOR ( 'NONE', #8319, 1000.000000000000000 ) ;
#5634=ORIENTED_EDGE ( 'NONE', *, *, #1380, .T. ) ;
#5636=EDGE_LOOP ( 'NONE', ( #6609, #9864, #656, #3753 ) ) ;
#5637=LINE ( 'NONE', #1425, #3203 ) ;
#5641=ORIENTED_EDGE ( 'NONE', *, *, #5275, .T. ) ;
#5644=AXIS2_PLACEMENT_3D ( 'NONE', #726, #3358, #4107 ) ;
#5645=ADVANCED_FACE ( 'NONE', ( #3006 ), #7950, .T. ) ;
#5649=ORIENTED_EDGE ( 'NONE', *, *, #6227, .F. ) ;
#5651=CARTESIAN_POINT ( 'NONE',  ( -6.145599950363623165, 19.66631150450993815, 3.355508642977428124 ) ) ;
#5657=ADVANCED_FACE ( 'NONE', ( #7128 ), #5418, .T. ) ;
#5667=FACE_OUTER_BOUND ( 'NONE', #5874, .T. ) ;
#5676=CARTESIAN_POINT ( 'NONE',  ( -3.785909150703094195, 19.34316356887878285, 5.890223162633836829 ) ) ;
#5678=AXIS2_PLACEMENT_3D ( 'NONE', #3495, #7761, #4462 ) ;
#5688=CIRCLE ( 'NONE', #9196, 4.500000000000000888 ) ;
#5697=AXIS2_PLACEMENT_3D ( 'NONE', #5776, #9087, #10811 ) ;
#5700=CARTESIAN_POINT ( 'NONE',  ( -0.5000000000000000000, 10.00000000000000355, 6.982120021884467675 ) ) ;
#5705=CARTESIAN_POINT ( 'NONE',  ( 0.1668442477450398642, 19.66631150450990617, -6.999999999999997335 ) ) ;
#5709=DIRECTION ( 'NONE',  ( -0.1889822365046156527, -0.000000000000000000, 0.9819805060619652970 ) ) ;
#5713=VERTEX_POINT ( 'NONE', #10539 ) ;
#5719=DIRECTION ( 'NONE',  ( 0.000000000000000000, 0.000000000000000000, 1.000000000000000000 ) ) ;
#5721=CARTESIAN_POINT ( 'NONE',  ( 0.000000000000000000, 10.00000000000000355, 0.000000000000000000 ) ) ;
#5725=VERTEX_POINT ( 'NONE', #4700 ) ;
#5728=ORIENTED_EDGE ( 'NONE', *, *, #10024, .T. ) ;
#5729=ADVANCED_FACE ( 'NONE', ( #3695 ), #6254, .T. ) ;
#5731=CARTESIAN_POINT ( 'NONE',  ( -3.500000000000049294, 20.00000000000000355, 6.062177826491040200 ) ) ;
#5738=LINE ( 'NONE', #8107, #5264 ) ;
#5747=DIRECTION ( 'NONE',  ( 0.9449111825230630535, -0.000000000000000000, 0.3273268353540027542 ) ) ;
#5750=LINE ( 'NONE', #9833, #2113 ) ;
#5751=( NAMED_UNIT ( * ) PLANE_ANGLE_UNIT ( ) SI_UNIT ( $, .RADIAN. ) );
#5761=VERTEX_POINT ( 'NONE', #2851 ) ;
#5762=CARTESIAN_POINT ( 'NONE',  ( 3.500000000000004885, 20.00000000000000355, -6.062177826491062405 ) ) ;
#5767=ORIENTED_EDGE ( 'NONE', *, *, #3696, .T. ) ;
#5776=CARTESIAN_POINT ( 'NONE',  ( -11.42163336986822308, 7.781088913245559624, -7.171633369868438912 ) ) ;
#5780=CYLINDRICAL_SURFACE ( 'NONE', #2506, 2.149999999999999911 ) ;
#5783=AXIS2_PLACEMENT_3D ( 'NONE', #6112, #4278, #6881 ) ;
#5786=EDGE_CURVE ( 'NONE', #9491, #7766, #10028, .T. ) ;
#5788=DIRECTION ( 'NONE',  ( 0.000000000000000000, 0.000000000000000000, -1.000000000000000000 ) ) ;
#5789=ORIENTED_EDGE ( 'NONE', *, *, #3481, .T. ) ;
#5791=SHAPE_DEFINITION_REPRESENTATION ( #2896, #6555 ) ;
#5795=PLANE ( 'NONE',  #7452 ) ;
#5807=FILL_AREA_STYLE ('',( #8280 ) ) ;
#5816=AXIS2_PLACEMENT_3D ( 'NONE', #378, #10537, #277 ) ;
#5819=ADVANCED_FACE ( 'NONE', ( #6456 ), #5780, .F. ) ;
#5833=VECTOR ( 'NONE', #8187, 1000.000000000000114 ) ;
#5836=DIRECTION ( 'NONE',  ( 0.000000000000000000, -1.000000000000000000, 0.000000000000000000 ) ) ;
#5841=DIRECTION ( 'NONE',  ( 0.000000000000000000, 0.000000000000000000, -1.000000000000000000 ) ) ;
#5842=CARTESIAN_POINT ( 'NONE',  ( 10.81217782649105708, 10.00000000000000355, 5.665063509461154112 ) ) ;
#5843=VECTOR ( 'NONE', #2026, 1000.000000000000000 ) ;
#5844=CARTESIAN_POINT ( 'NONE',  ( -5.796693311223946488, 19.03096903053430466, 3.924072712834398846 ) ) ;
#5847=DIRECTION ( 'NONE',  ( -0.8660254037844328234, 0.000000000000000000, -0.5000000000000101030 ) ) ;
#5849=EDGE_CURVE ( 'NONE', #5164, #1247, #583, .T. ) ;
#5862=VERTEX_POINT ( 'NONE', #2614 ) ;
#5863=ADVANCED_FACE ( 'NONE', ( #10320 ), #1638, .T. ) ;
#5872=VECTOR ( 'NONE', #8298, 1000.000000000000000 ) ;
#5874=EDGE_LOOP ( 'NONE', ( #3444, #4361, #9148 ) ) ;
#5882=AXIS2_PLACEMENT_3D ( 'NONE', #6196, #280, #8882 ) ;
#5896=DIRECTION ( 'NONE',  ( -3.491481338843133355E-15, 0.000000000000000000, 1.000000000000000000 ) ) ;
#5899=DIRECTION ( 'NONE',  ( 0.4330127018922207971, -0.8660254037844380415, -0.2499999999999995282 ) ) ;
#5902=DIRECTION ( 'NONE',  ( 0.000000000000000000, 0.000000000000000000, 1.000000000000000000 ) ) ;
#5905=CARTESIAN_POINT ( 'NONE',  ( 12.19615242270663735, 10.00000000000000355, -0.4999999999999575340 ) ) ;
#5914=EDGE_CURVE ( 'NONE', #10217, #3157, #10257, .T. ) ;
#5921=ADVANCED_FACE ( 'NONE', ( #10144 ), #6838, .T. ) ;
#5924=CARTESIAN_POINT ( 'NONE',  ( -0.5000000000000000000, 7.781088913245555183, -13.47724133595216500 ) ) ;
#5926=ORIENTED_EDGE ( 'NONE', *, *, #5227, .F. ) ;
#5936=VERTEX_POINT ( 'NONE', #5127 ) ;
#5958=PLANE ( 'NONE',  #7616 ) ;
#5962=FACE_BOUND ( 'NONE', #4715, .T. ) ;
#5973=DIRECTION ( 'NONE',  ( -0.3061862178478914065, -0.3535533905932741194, -0.8838834764831863255 ) ) ;
#5975=ORIENTED_EDGE ( 'NONE', *, *, #2086, .F. ) ;
#5976=CARTESIAN_POINT ( 'NONE',  ( 0.000000000000000000, 10.10000000000000497, -4.500000000000000888 ) ) ;
#5984=ORIENTED_EDGE ( 'NONE', *, *, #10507, .F. ) ;
#5994=PLANE ( 'NONE',  #5783 ) ;
#5998=CARTESIAN_POINT ( 'NONE',  ( 0.5000000000000000000, 7.781088913245554295, -13.47724133595216323 ) ) ;
#6008=PLANE ( 'NONE',  #595 ) ;
#6015=ORIENTED_EDGE ( 'NONE', *, *, #4702, .T. ) ;
#6017=AXIS2_PLACEMENT_3D ( 'NONE', #8595, #7065, #10199 ) ;
#6025=DIRECTION ( 'NONE',  ( -0.000000000000000000, 1.000000000000000000, -0.000000000000000000 ) ) ;
#6027=AXIS2_PLACEMENT_3D ( 'NONE', #8031, #8131, #3944 ) ;
#6048=LINE ( 'NONE', #6161, #3030 ) ;
#6056=CARTESIAN_POINT ( 'NONE',  ( 6.531088913245547189, 10.00000000000000355, -10.31217782649106240 ) ) ;
#6061=EDGE_CURVE ( 'NONE', #9255, #7282, #9544, .T. ) ;
#6064=CIRCLE ( 'NONE', #9750, 6.999999999999997335 ) ;
#6066=ADVANCED_FACE ( 'NONE', ( #2838 ), #9487, .T. ) ;
#6072=CARTESIAN_POINT ( 'NONE',  ( -5.978755702618506085, 19.66631150450992394, -3.644491357022579425 ) ) ;
#6074=CARTESIAN_POINT ( 'NONE',  ( 6.296693311223896750, 19.03096903053431177, 3.058047309050043960 ) ) ;
#6078=EDGE_LOOP ( 'NONE', ( #3053, #5531, #2314, #1626 ) ) ;
#6081=ORIENTED_EDGE ( 'NONE', *, *, #26, .F. ) ;
#6088=DIRECTION ( 'NONE',  ( 0.000000000000000000, 0.000000000000000000, 1.000000000000000000 ) ) ;
#6096=ORIENTED_EDGE ( 'NONE', *, *, #2086, .T. ) ;
#6112=CARTESIAN_POINT ( 'NONE',  ( 0.000000000000000000, 10.00000000000000355, 0.000000000000000000 ) ) ;
#6113=CARTESIAN_POINT ( 'NONE',  ( 6.062177826491077504, 20.00000000000000355, -3.499999999999985345 ) ) ;
#6114=PLANE ( 'NONE',  #2313 ) ;
#6115=DIRECTION ( 'NONE',  ( 0.000000000000000000, -1.000000000000000000, 0.000000000000000000 ) ) ;
#6116=DIRECTION ( 'NONE',  ( -0.9449111825230702699, -0.000000000000000000, 0.3273268353539822706 ) ) ;
#6122=DIRECTION ( 'NONE',  ( 0.4330127018922192428, -0.8660254037844380415, 0.2500000000000026645 ) ) ;
#6137=DIRECTION ( 'NONE',  ( 0.000000000000000000, 0.000000000000000000, 1.000000000000000000 ) ) ;
#6140=EDGE_LOOP ( 'NONE', ( #9261, #3261, #7231 ) ) ;
#6146=ORIENTED_EDGE ( 'NONE', *, *, #1867, .T. ) ;
#6153=VECTOR ( 'NONE', #6189, 1000.000000000000114 ) ;
#6161=CARTESIAN_POINT ( 'NONE',  ( -0.1339745962155587111, 10.00000000000000355, -12.92820323027550700 ) ) ;
#6165=CARTESIAN_POINT ( 'NONE',  ( 3.208128317448934119, 19.34316356887880772, -6.223805082245734255 ) ) ;
#6177=CARTESIAN_POINT ( 'NONE',  ( 0.000000000000000000, 20.00000000000000355, 0.000000000000000000 ) ) ;
#6178=DIRECTION ( 'NONE',  ( 0.9819805060619657411, -0.000000000000000000, 0.1889822365046139596 ) ) ;
#6179=CARTESIAN_POINT ( 'NONE',  ( 2.850480947161637246, 19.75000000000000711, 5.937177826491089050 ) ) ;
#6183=ORIENTED_EDGE ( 'NONE', *, *, #688, .T. ) ;
#6189=DIRECTION ( 'NONE',  ( 0.2500000000000010547, -0.8660254037844380415, -0.4330127018922199089 ) ) ;
#6191=ORIENTED_EDGE ( 'NONE', *, *, #5275, .F. ) ;
#6196=CARTESIAN_POINT ( 'NONE',  ( 0.000000000000000000, 10.00000000000000355, 0.000000000000000000 ) ) ;
#6203=CARTESIAN_POINT ( 'NONE',  ( 0.000000000000000000, 7.000000000000003553, -4.500000000000000888 ) ) ;
#6207=DIRECTION ( 'NONE',  ( 0.000000000000000000, 0.000000000000000000, 1.000000000000000000 ) ) ;
#6208=DIRECTION ( 'NONE',  ( 0.000000000000000000, 1.000000000000000000, 0.000000000000000000 ) ) ;
#6227=EDGE_CURVE ( 'NONE', #824, #8414, #9219, .T. ) ;
#6229=CARTESIAN_POINT ( 'NONE',  ( -3.058047309049933382, 10.00000000000000355, -6.296693311223948264 ) ) ;
#6233=DIRECTION ( 'NONE',  ( -0.000000000000000000, -1.000000000000000000, -0.000000000000000000 ) ) ;
#6235=DIRECTION ( 'NONE',  ( 0.000000000000000000, 1.000000000000000000, 0.000000000000000000 ) ) ;
#6242=DIRECTION ( 'NONE',  ( 0.000000000000000000, -0.000000000000000000, 1.000000000000000000 ) ) ;
#6243=CARTESIAN_POINT ( 'NONE',  ( 13.47724133595215790, 7.781088913245551630, 0.5000000000000470735 ) ) ;
#6245=AXIS2_PLACEMENT_3D ( 'NONE', #2668, #6235, #10254 ) ;
#6254=CYLINDRICAL_SURFACE ( 'NONE', #5882, 6.999999999999997335 ) ;
#6255=ORIENTED_EDGE ( 'NONE', *, *, #3696, .F. ) ;
#6257=CARTESIAN_POINT ( 'NONE',  ( 0.000000000000000000, 10.00000000000000355, 0.000000000000000000 ) ) ;
#6261=LINE ( 'NONE', #8015, #5466 ) ;
#6270=ORIENTED_EDGE ( 'NONE', *, *, #4733, .T. ) ;
#6271=EDGE_CURVE ( 'NONE', #2551, #1630, #9362, .T. ) ;
#6279=DIRECTION ( 'NONE',  ( 0.000000000000000000, 0.000000000000000000, -1.000000000000000000 ) ) ;
#6282=ORIENTED_EDGE ( 'NONE', *, *, #7446, .F. ) ;
#6290=CARTESIAN_POINT ( 'NONE',  ( 0.000000000000000000, 10.00000000000000355, 0.000000000000000000 ) ) ;
#6293=VERTEX_POINT ( 'NONE', #7086 ) ;
#6296=CARTESIAN_POINT ( 'NONE',  ( 0.4330127018922207971, 0.000000000000000000, -0.2499999999999974465 ) ) ;
#6307=CARTESIAN_POINT ( 'NONE',  ( 2.632990618166809235E-16, 10.10000000000000497, 2.149999999999999911 ) ) ;
#6313=EDGE_LOOP ( 'NONE', ( #8660, #2152, #3332, #3065, #102, #3656 ) ) ;
#6314=AXIS2_PLACEMENT_3D ( 'NONE', #9846, #2791, #8144 ) ;
#6315=DIRECTION ( 'NONE',  ( 0.000000000000000000, 1.000000000000000000, 0.000000000000000000 ) ) ;
#6325=PLANE ( 'NONE',  #8674 ) ;
#6334=CYLINDRICAL_SURFACE ( 'NONE', #9830, 2.149999999999999911 ) ;
#6336=EDGE_CURVE ( 'NONE', #6450, #6764, #2699, .T. ) ;
#6339=DIRECTION ( 'NONE',  ( 0.000000000000000000, 0.000000000000000000, 1.000000000000000000 ) ) ;
#6341=CARTESIAN_POINT ( 'NONE',  ( 11.26313972081439196, 10.00000000000000355, 6.348076211353378184 ) ) ;
#6346=ORIENTED_EDGE ( 'NONE', *, *, #6403, .T. ) ;
#6351=DIRECTION ( 'NONE',  ( 0.000000000000000000, 0.000000000000000000, 1.000000000000000000 ) ) ;
#6354=ORIENTED_EDGE ( 'NONE', *, *, #2748, .T. ) ;
#6360=VECTOR ( 'NONE', #5049, 1000.000000000000114 ) ;
#6363=DIRECTION ( 'NONE',  ( -0.5000000000000009992, -0.8660254037844380415, -5.237222008264710288E-15 ) ) ;
#6380=AXIS2_PLACEMENT_3D ( 'NONE', #1137, #6315, #4617 ) ;
#6381=VECTOR ( 'NONE', #4185, 1000.000000000000000 ) ;
#6386=ORIENTED_EDGE ( 'NONE', *, *, #8359, .T. ) ;
#6388=ORIENTED_EDGE ( 'NONE', *, *, #478, .F. ) ;
#6390=CIRCLE ( 'NONE', #10440, 4.500000000000000888 ) ;
#6393=DIRECTION ( 'NONE',  ( -0.1889822365046077146, 0.000000000000000000, -0.9819805060619668513 ) ) ;
#6394=DIRECTION ( 'NONE',  ( 0.5000000000000009992, 0.000000000000000000, -0.8660254037844380415 ) ) ;
#6401=CIRCLE ( 'NONE', #3741, 12.77350269189627063 ) ;
#6403=EDGE_CURVE ( 'NONE', #7845, #8513, #6401, .T. ) ;
#6407=( BOUNDED_CURVE ( )  B_SPLINE_CURVE ( 3, ( #4586, #7934, #6072, #8593 ),
 .UNSPECIFIED., .F., .F. ) 
 B_SPLINE_CURVE_WITH_KNOTS ( ( 4, 4 ),
 ( 3.927175151554401999, 3.998664601439922528 ),
 .UNSPECIFIED. ) 
 CURVE ( )  GEOMETRIC_REPRESENTATION_ITEM ( )  RATIONAL_B_SPLINE_CURVE ( ( 1.000000000000000000, 0.9995741502243209453, 0.9995741502243209453, 1.000000000000000000 ) ) 
 REPRESENTATION_ITEM ( '' )  );
#6409=VECTOR ( 'NONE', #3324, 1000.000000000000000 ) ;
#6410=AXIS2_PLACEMENT_3D ( 'NONE', #2194, #5571, #1266 ) ;
#6413=ORIENTED_EDGE ( 'NONE', *, *, #9507, .F. ) ;
#6416=DIRECTION ( 'NONE',  ( 0.000000000000000000, -0.8660254037844380415, 0.5000000000000009992 ) ) ;
#6418=CARTESIAN_POINT ( 'NONE',  ( 6.062177826491077504, 20.00000000000000355, -3.499999999999985345 ) ) ;
#6428=AXIS2_PLACEMENT_3D ( 'NONE', #1475, #4858, #8203 ) ;
#6435=DIRECTION ( 'NONE',  ( -0.4330127018922226845, -0.8660254037844380415, 0.2499999999999965306 ) ) ;
#6438=VERTEX_POINT ( 'NONE', #5905 ) ;
#6442=DIRECTION ( 'NONE',  ( -0.8660254037844432595, 0.000000000000000000, 0.4999999999999919509 ) ) ;
#6445=DIRECTION ( 'NONE',  ( -0.000000000000000000, 1.000000000000000000, -0.000000000000000000 ) ) ;
#6446=CARTESIAN_POINT ( 'NONE',  ( 0.5000000000000000000, 0.000000000000000000, 0.000000000000000000 ) ) ;
#6447=DIRECTION ( 'NONE',  ( 0.000000000000000000, 0.8660254037844380415, 0.5000000000000009992 ) ) ;
#6448=VERTEX_POINT ( 'NONE', #5844 ) ;
#6450=VERTEX_POINT ( 'NONE', #2513 ) ;
#6456=FACE_OUTER_BOUND ( 'NONE', #4819, .T. ) ;
#6457=LINE ( 'NONE', #2238, #1627 ) ;
#6458=EDGE_CURVE ( 'NONE', #7784, #6293, #9574, .T. ) ;
#6459=EDGE_LOOP ( 'NONE', ( #5789, #6473 ) ) ;
#6464=ADVANCED_FACE ( 'NONE', ( #1647 ), #5958, .F. ) ;
#6467=ORIENTED_EDGE ( 'NONE', *, *, #1129, .F. ) ;
#6473=ORIENTED_EDGE ( 'NONE', *, *, #5262, .T. ) ;
#6479=CARTESIAN_POINT ( 'NONE',  ( -6.994037468151967474, 19.34316356887880062, -0.3335819196119432228 ) ) ;
#6480=LINE ( 'NONE', #2269, #2291 ) ;
#6482=LINE ( 'NONE', #4725, #1977 ) ;
#6483=EDGE_CURVE ( 'NONE', #7391, #1515, #984, .T. ) ;
#6485=EDGE_LOOP ( 'NONE', ( #9572, #6718, #7501, #7768, #1286, #5117, #4060, #8963, #9790 ) ) ;
#6486=ORIENTED_EDGE ( 'NONE', *, *, #5459, .T. ) ;
#6490=DIRECTION ( 'NONE',  ( 0.000000000000000000, 1.000000000000000000, 0.000000000000000000 ) ) ;
#6491=CARTESIAN_POINT ( 'NONE',  ( -12.19615242270664979, 10.00000000000000355, 0.4999999999998722688 ) ) ;
#6501=CARTESIAN_POINT ( 'NONE',  ( -3.924072712834500543, 19.03096903053431177, 5.796693311223878098 ) ) ;
#6507=EDGE_CURVE ( 'NONE', #5936, #3864, #5688, .T. ) ;
#6519=ORIENTED_EDGE ( 'NONE', *, *, #6530, .F. ) ;
#6521=ADVANCED_FACE ( 'NONE', ( #3057 ), #1472, .F. ) ;
#6530=EDGE_CURVE ( 'NONE', #6764, #6584, #2947, .T. ) ;
#6531=CARTESIAN_POINT ( 'NONE',  ( 3.499999999999957812, 20.00000000000000355, 6.062177826491091714 ) ) ;
#6536=ADVANCED_FACE ( 'NONE', ( #7267 ), #4643, .F. ) ;
#6544=ORIENTED_EDGE ( 'NONE', *, *, #2029, .T. ) ;
#6551=ORIENTED_EDGE ( 'NONE', *, *, #6483, .F. ) ;
#6553=ORIENTED_EDGE ( 'NONE', *, *, #4410, .T. ) ;
#6555=SHAPE_REPRESENTATION ( 'Inner Conical Burr Core', ( #7040 ), #1019 ) ;
#6556=LINE ( 'NONE', #692, #10117 ) ;
#6557=CARTESIAN_POINT ( 'NONE',  ( -6.999999999999997335, 20.00000000000000355, -6.917209860457518289E-14 ) ) ;
#6567=VECTOR ( 'NONE', #1517, 1000.000000000000000 ) ;
#6574=AXIS2_PLACEMENT_3D ( 'NONE', #4892, #1510, #3050 ) ;
#6584=VERTEX_POINT ( 'NONE', #9756 ) ;
#6591=DIRECTION ( 'NONE',  ( 0.000000000000000000, 0.000000000000000000, 1.000000000000000000 ) ) ;
#6592=CARTESIAN_POINT ( 'NONE',  ( -13.47724133595216678, 7.781088913245558736, -0.5000000000001412204 ) ) ;
#6593=AXIS2_PLACEMENT_3D ( 'NONE', #9369, #6787, #8423 ) ;
#6595=ORIENTED_EDGE ( 'NONE', *, *, #9720, .T. ) ;
#6601=CARTESIAN_POINT ( 'NONE',  ( 6.296693311223896750, 10.00000000000000355, 3.058047309050043960 ) ) ;
#6603=DIRECTION ( 'NONE',  ( 0.000000000000000000, 0.000000000000000000, 1.000000000000000000 ) ) ;
#6607=EDGE_LOOP ( 'NONE', ( #9317, #1122, #7593, #5027 ) ) ;
#6609=ORIENTED_EDGE ( 'NONE', *, *, #2573, .F. ) ;
#6612=FACE_OUTER_BOUND ( 'NONE', #6703, .T. ) ;
#6616=PLANE ( 'NONE',  #10276 ) ;
#6625=CARTESIAN_POINT ( 'NONE',  ( 0.000000000000000000, 7.000000000000003553, 0.000000000000000000 ) ) ;
#6626=ORIENTED_EDGE ( 'NONE', *, *, #9810, .F. ) ;
#6629=ORIENTED_EDGE ( 'NONE', *, *, #8957, .T. ) ;
#6638=SURFACE_SIDE_STYLE ('',( #9945 ) ) ;
#6639=FACE_OUTER_BOUND ( 'NONE', #3560, .T. ) ;
#6640=DIRECTION ( 'NONE',  ( 0.000000000000000000, 1.000000000000000000, 0.000000000000000000 ) ) ;
#6650=PLANE ( 'NONE',  #153 ) ;
#6651=ORIENTED_EDGE ( 'NONE', *, *, #8484, .F. ) ;
#6678=ADVANCED_FACE ( 'NONE', ( #10536 ), #10080, .T. ) ;
#6683=ADVANCED_FACE ( 'NONE', ( #6612 ), #9139, .T. ) ;
#6689=ORIENTED_EDGE ( 'NONE', *, *, #10507, .T. ) ;
#6690=( BOUNDED_CURVE ( )  B_SPLINE_CURVE ( 3, ( #2319, #2424, #5705, #9112 ),
 .UNSPECIFIED., .F., .F. ) 
 B_SPLINE_CURVE_WITH_KNOTS ( ( 4, 4 ),
 ( 3.927175151554402888, 3.998664601439924304 ),
 .UNSPECIFIED. ) 
 CURVE ( )  GEOMETRIC_REPRESENTATION_ITEM ( )  RATIONAL_B_SPLINE_CURVE ( ( 1.000000000000000000, 0.9995741502243209453, 0.9995741502243209453, 1.000000000000000000 ) ) 
 REPRESENTATION_ITEM ( '' )  );
#6697=ORIENTED_EDGE ( 'NONE', *, *, #5257, .F. ) ;
#6701=DIRECTION ( 'NONE',  ( -0.2499999999999950318, -0.8660254037844380415, -0.4330127018922234061 ) ) ;
#6703=EDGE_LOOP ( 'NONE', ( #2416, #4551, #1560, #9060 ) ) ;
#6709=LINE ( 'NONE', #2279, #10781 ) ;
#6711=VECTOR ( 'NONE', #4813, 1000.000000000000000 ) ;
#6718=ORIENTED_EDGE ( 'NONE', *, *, #10848, .T. ) ;
#6731=EDGE_CURVE ( 'NONE', #9293, #399, #401, .T. ) ;
#6732=ADVANCED_FACE ( 'NONE', ( #8420 ), #691, .F. ) ;
#6736=CARTESIAN_POINT ( 'NONE',  ( -0.3335819196118703922, 19.34316356887877220, 6.994037468151971026 ) ) ;
#6742=EDGE_LOOP ( 'NONE', ( #1258, #7408, #4137, #6386 ) ) ;
#6748=CARTESIAN_POINT ( 'NONE',  ( -3.500000000000040412, 20.00000000000000355, 6.062177826491044641 ) ) ;
#6752=SURFACE_SIDE_STYLE ('',( #10054 ) ) ;
#6762=ORIENTED_EDGE ( 'NONE', *, *, #6868, .T. ) ;
#6764=VERTEX_POINT ( 'NONE', #2397 ) ;
#6766=CARTESIAN_POINT ( 'NONE',  ( 5.796693311223918066, 19.03096903053432598, -3.924072712834439702 ) ) ;
#6770=LINE ( 'NONE', #7579, #2775 ) ;
#6778=DIRECTION ( 'NONE',  ( 0.5000000000000009992, 0.000000000000000000, -0.8660254037844380415 ) ) ;
#6781=AXIS2_PLACEMENT_3D ( 'NONE', #10082, #2670, #3325 ) ;
#6784=DIRECTION ( 'NONE',  ( 1.000000000000000000, 0.000000000000000000, 3.491481338843133355E-15 ) ) ;
#6787=DIRECTION ( 'NONE',  ( 0.000000000000000000, 1.000000000000000000, 0.000000000000000000 ) ) ;
#6788=CARTESIAN_POINT ( 'NONE',  ( 6.062177826491054411, 20.00000000000000355, 3.500000000000023981 ) ) ;
#6793=CARTESIAN_POINT ( 'NONE',  ( 0.000000000000000000, 20.00000000000000355, 0.000000000000000000 ) ) ;
#6797=CARTESIAN_POINT ( 'NONE',  ( 1.214306433183764808E-14, 10.00000000000000355, 12.77350269189627063 ) ) ;
#6824=EDGE_CURVE ( 'NONE', #978, #9763, #1635, .T. ) ;
#6829=ORIENTED_EDGE ( 'NONE', *, *, #6731, .T. ) ;
#6837=DIRECTION ( 'NONE',  ( -0.000000000000000000, 1.000000000000000000, -0.000000000000000000 ) ) ;
#6838=PLANE ( 'NONE',  #7641 ) ;
#6839=FACE_OUTER_BOUND ( 'NONE', #8673, .T. ) ;
#6844=CARTESIAN_POINT ( 'NONE',  ( -0.1668442477450398642, 19.66631150450990617, 6.999999999999997335 ) ) ;
#6849=VECTOR ( 'NONE', #4753, 1000.000000000000000 ) ;
#6854=EDGE_CURVE ( 'NONE', #2965, #5862, #4900, .T. ) ;
#6855=CIRCLE ( 'NONE', #9840, 6.999999999999997335 ) ;
#6861=ORIENTED_EDGE ( 'NONE', *, *, #10533, .T. ) ;
#6868=EDGE_CURVE ( 'NONE', #1630, #10532, #7060, .T. ) ;
#6875=DIRECTION ( 'NONE',  ( -0.2499999999999950318, -0.8660254037844380415, -0.4330127018922235171 ) ) ;
#6881=DIRECTION ( 'NONE',  ( 0.000000000000000000, -0.000000000000000000, 1.000000000000000000 ) ) ;
#6886=CARTESIAN_POINT ( 'NONE',  ( 0.000000000000000000, 10.10000000000000497, -2.149999999999999911 ) ) ;
#6897=CARTESIAN_POINT ( 'NONE',  ( 5.665063509461043978, 10.00000000000000355, 10.81217782649112102 ) ) ;
#6901=DIRECTION ( 'NONE',  ( 0.000000000000000000, -1.000000000000000000, 0.000000000000000000 ) ) ;
#6902=DIRECTION ( 'NONE',  ( 0.000000000000000000, 0.000000000000000000, -1.000000000000000000 ) ) ;
#6918=CARTESIAN_POINT ( 'NONE',  ( 0.000000000000000000, 10.00000000000000355, 0.000000000000000000 ) ) ;
#6919=CYLINDRICAL_SURFACE ( 'NONE', #10293, 6.999999999999997335 ) ;
#6929=DIRECTION ( 'NONE',  ( 0.2499999999999979461, -0.8660254037844380415, 0.4330127018922216853 ) ) ;
#6934=VERTEX_POINT ( 'NONE', #6897 ) ;
#6938=VECTOR ( 'NONE', #6447, 1000.000000000000000 ) ;
#6948=DIRECTION ( 'NONE',  ( -0.4999999999999888423, 0.000000000000000000, -0.8660254037844449249 ) ) ;
#6951=VECTOR ( 'NONE', #185, 1000.000000000000000 ) ;
#6953=EDGE_LOOP ( 'NONE', ( #1989, #4287, #3630, #2362 ) ) ;
#6961=CARTESIAN_POINT ( 'NONE',  ( 0.000000000000000000, 10.00000000000000355, 0.000000000000000000 ) ) ;
#6966=ADVANCED_FACE ( 'NONE', ( #7008 ), #8535, .T. ) ;
#6968=AXIS2_PLACEMENT_3D ( 'NONE', #221, #7905, #7947 ) ;
#6969=ORIENTED_EDGE ( 'NONE', *, *, #10167, .F. ) ;
#6971=DIRECTION ( 'NONE',  ( 0.000000000000000000, 0.000000000000000000, 1.000000000000000000 ) ) ;
#6977=CYLINDRICAL_SURFACE ( 'NONE', #4655, 6.999999999999997335 ) ;
#6981=CARTESIAN_POINT ( 'NONE',  ( 12.77350269189627063, 10.00000000000000355, 3.256982943917019352E-14 ) ) ;
#7000=LINE ( 'NONE', #2828, #2498 ) ;
#7008=FACE_OUTER_BOUND ( 'NONE', #3574, .T. ) ;
#7011=CARTESIAN_POINT ( 'NONE',  ( 0.000000000000000000, 10.00000000000000355, 0.000000000000000000 ) ) ;
#7016=EDGE_CURVE ( 'NONE', #1515, #9174, #7639, .T. ) ;
#7020=DIRECTION ( 'NONE',  ( 1.000000000000000000, 0.000000000000000000, 3.491481338843133355E-15 ) ) ;
#7022=ORIENTED_EDGE ( 'NONE', *, *, #7252, .F. ) ;
#7029=CARTESIAN_POINT ( 'NONE',  ( 3.058047309049978235, 10.00000000000000355, 6.296693311223928724 ) ) ;
#7034=DIRECTION ( 'NONE',  ( -0.4999999999999919509, 0.000000000000000000, -0.8660254037844432595 ) ) ;
#7040=AXIS2_PLACEMENT_3D ( 'NONE', #1904, #3431, #7048 ) ;
#7048=DIRECTION ( 'NONE',  ( 1.000000000000000000, 0.000000000000000000, 0.000000000000000000 ) ) ;
#7049=PLANE ( 'NONE',  #2081 ) ;
#7050=MANIFOLD_SOLID_BREP ( 'AdvancedHole1', #4380 ) ;
#7060=LINE ( 'NONE', #1155, #3025 ) ;
#7065=DIRECTION ( 'NONE',  ( 0.000000000000000000, 1.000000000000000000, 0.000000000000000000 ) ) ;
#7067=DIRECTION ( 'NONE',  ( 0.8660254037844397068, 0.000000000000000000, -0.4999999999999979461 ) ) ;
#7078=AXIS2_PLACEMENT_3D ( 'NONE', #4248, #8606, #4425 ) ;
#7079=AXIS2_PLACEMENT_3D ( 'NONE', #9686, #8130, #2110 ) ;
#7082=AXIS2_PLACEMENT_3D ( 'NONE', #6446, #10637, #3795 ) ;
#7086=CARTESIAN_POINT ( 'NONE',  ( -12.77350269189627063, 10.00000000000000355, -1.344410693882025246E-13 ) ) ;
#7091=DIRECTION ( 'NONE',  ( 0.000000000000000000, 0.000000000000000000, 1.000000000000000000 ) ) ;
#7103=DIRECTION ( 'NONE',  ( 0.3273268353539987574, 0.000000000000000000, -0.9449111825230646078 ) ) ;
#7104=CARTESIAN_POINT ( 'NONE',  ( -0.4330127018922207971, 0.000000000000000000, 0.2499999999999974465 ) ) ;
#7108=ORIENTED_EDGE ( 'NONE', *, *, #6824, .F. ) ;
#7113=DIRECTION ( 'NONE',  ( 0.4330127018922207971, -0.8660254037844380415, -0.2499999999999995282 ) ) ;
#7114=CIRCLE ( 'NONE', #2329, 12.77350269189627063 ) ;
#7115=CARTESIAN_POINT ( 'NONE',  ( -0.2499999999999990286, 0.000000000000000000, -0.4330127018922199644 ) ) ;
#7116=AXIS2_PLACEMENT_3D ( 'NONE', #9919, #594, #1364 ) ;
#7118=PLANE ( 'NONE',  #9741 ) ;
#7120=ORIENTED_EDGE ( 'NONE', *, *, #7810, .F. ) ;
#7127=CARTESIAN_POINT ( 'NONE',  ( 7.171633369868234631, 7.781088913245556959, 11.42163336986834388 ) ) ;
#7128=FACE_OUTER_BOUND ( 'NONE', #6078, .T. ) ;
#7138=AXIS2_PLACEMENT_3D ( 'NONE', #1362, #8158, #5512 ) ;
#7149=CARTESIAN_POINT ( 'NONE',  ( -0.3335819196118727237, 19.34316356887877930, -6.994037468151971026 ) ) ;
#7161=ORIENTED_EDGE ( 'NONE', *, *, #3435, .F. ) ;
#7178=EDGE_LOOP ( 'NONE', ( #6467, #5505, #4751, #5767, #1326, #10283 ) ) ;
#7202=CARTESIAN_POINT ( 'NONE',  ( 11.06217782649105175, 10.00000000000000355, 6.386751345948189496 ) ) ;
#7213=PLANE ( 'NONE',  #7082 ) ;
#7217=CARTESIAN_POINT ( 'NONE',  ( 12.92820323027550700, 10.00000000000000355, -0.1339745962155138304 ) ) ;
#7219=CARTESIAN_POINT ( 'NONE',  ( 4.946152422706616036, 10.00000000000000355, 3.433012701892241836 ) ) ;
#7223=EDGE_LOOP ( 'NONE', ( #9472, #1700, #9167, #3806, #9777, #6270 ) ) ;
#7226=DIRECTION ( 'NONE',  ( -0.4999999999999888423, 0.000000000000000000, -0.8660254037844449249 ) ) ;
#7231=ORIENTED_EDGE ( 'NONE', *, *, #9421, .F. ) ;
#7233=LINE ( 'NONE', #8897, #664 ) ;
#7239=ORIENTED_EDGE ( 'NONE', *, *, #1147, .F. ) ;
#7252=EDGE_CURVE ( 'NONE', #417, #10229, #6064, .T. ) ;
#7253=AXIS2_PLACEMENT_3D ( 'NONE', #8698, #3553, #10355 ) ;
#7260=PLANE ( 'NONE',  #8831 ) ;
#7261=LINE ( 'NONE', #4739, #9039 ) ;
#7263=ORIENTED_EDGE ( 'NONE', *, *, #2241, .F. ) ;
#7267=FACE_OUTER_BOUND ( 'NONE', #3559, .T. ) ;
#7269=EDGE_CURVE ( 'NONE', #6293, #8354, #10292, .T. ) ;
#7271=DIRECTION ( 'NONE',  ( 0.000000000000000000, 1.000000000000000000, 0.000000000000000000 ) ) ;
#7279=CARTESIAN_POINT ( 'NONE',  ( -6.062177826491100596, 20.00000000000000355, 3.499999999999942712 ) ) ;
#7282=VERTEX_POINT ( 'NONE', #10449 ) ;
#7291=EDGE_LOOP ( 'NONE', ( #1184, #6081, #6697, #9465 ) ) ;
#7293=VECTOR ( 'NONE', #3004, 999.9999999999998863 ) ;
#7303=VERTEX_POINT ( 'NONE', #6307 ) ;
#7309=DIRECTION ( 'NONE',  ( -0.4330127018922192428, 0.8660254037844380415, -0.2500000000000026645 ) ) ;
#7310=ADVANCED_FACE ( 'NONE', ( #7915 ), #343, .T. ) ;
#7319=EDGE_CURVE ( 'NONE', #1247, #5192, #2053, .T. ) ;
#7324=ORIENTED_EDGE ( 'NONE', *, *, #2666, .T. ) ;
#7326=EDGE_LOOP ( 'NONE', ( #8072, #1333, #5649 ) ) ;
#7335=DIRECTION ( 'NONE',  ( -0.7559289460184509535, -0.000000000000000000, -0.6546536707079810835 ) ) ;
#7340=ORIENTED_EDGE ( 'NONE', *, *, #4770, .T. ) ;
#7353=ORIENTED_EDGE ( 'NONE', *, *, #6061, .T. ) ;
#7354=ORIENTED_EDGE ( 'NONE', *, *, #5259, .F. ) ;
#7383=CARTESIAN_POINT ( 'NONE',  ( 6.999999999999997335, 20.00000000000000355, 3.024924061234557371E-14 ) ) ;
#7387=FACE_OUTER_BOUND ( 'NONE', #5143, .T. ) ;
#7391=VERTEX_POINT ( 'NONE', #1373 ) ;
#7402=LINE ( 'NONE', #1606, #7984 ) ;
#7404=EDGE_CURVE ( 'NONE', #6450, #10325, #276, .T. ) ;
#7406=CIRCLE ( 'NONE', #2630, 2.149999999999999911 ) ;
#7407=FACE_OUTER_BOUND ( 'NONE', #6742, .T. ) ;
#7408=ORIENTED_EDGE ( 'NONE', *, *, #7904, .F. ) ;
#7415=LINE ( 'NONE', #9235, #4911 ) ;
#7424=ORIENTED_EDGE ( 'NONE', *, *, #2873, .T. ) ;
#7430=AXIS2_PLACEMENT_3D ( 'NONE', #3804, #3537, #6351 ) ;
#7438=DIRECTION ( 'NONE',  ( 0.000000000000000000, 1.000000000000000000, 0.000000000000000000 ) ) ;
#7446=EDGE_CURVE ( 'NONE', #399, #8513, #4086, .T. ) ;
#7452=AXIS2_PLACEMENT_3D ( 'NONE', #8328, #8267, #3075 ) ;
#7455=LINE ( 'NONE', #5592, #8286 ) ;
#7466=DIRECTION ( 'NONE',  ( 0.000000000000000000, 1.000000000000000000, 0.000000000000000000 ) ) ;
#7477=DIRECTION ( 'NONE',  ( 0.9449111825230666062, -0.000000000000000000, -0.3273268353539928177 ) ) ;
#7478=PLANE ( 'NONE',  #1073 ) ;
#7482=FACE_OUTER_BOUND ( 'NONE', #2394, .T. ) ;
#7484=ORIENTED_EDGE ( 'NONE', *, *, #5050, .T. ) ;
#7488=EDGE_CURVE ( 'NONE', #7766, #748, #3459, .T. ) ;
#7496=ORIENTED_EDGE ( 'NONE', *, *, #7749, .T. ) ;
#7501=ORIENTED_EDGE ( 'NONE', *, *, #6403, .F. ) ;
#7505=DIRECTION ( 'NONE',  ( 0.000000000000000000, 1.000000000000000000, 0.000000000000000000 ) ) ;
#7529=CARTESIAN_POINT ( 'NONE',  ( 3.924072712834459686, 19.03096903053429756, -5.796693311223905631 ) ) ;
#7532=DIRECTION ( 'NONE',  ( 1.000000000000000000, 0.000000000000000000, -0.000000000000000000 ) ) ;
#7534=ORIENTED_EDGE ( 'NONE', *, *, #5227, .T. ) ;
#7541=DIRECTION ( 'NONE',  ( 0.000000000000000000, 0.000000000000000000, 1.000000000000000000 ) ) ;
#7543=DIRECTION ( 'NONE',  ( -0.4999999999999888423, 0.000000000000000000, -0.8660254037844449249 ) ) ;
#7551=LINE ( 'NONE', #10090, #2998 ) ;
#7553=ORIENTED_EDGE ( 'NONE', *, *, #9356, .F. ) ;
#7558=AXIS2_PLACEMENT_3D ( 'NONE', #3589, #3644, #10336 ) ;
#7560=EDGE_LOOP ( 'NONE', ( #1925, #7263, #1721, #3814 ) ) ;
#7561=FACE_OUTER_BOUND ( 'NONE', #7867, .T. ) ;
#7566=( LENGTH_UNIT ( ) NAMED_UNIT ( * ) SI_UNIT ( .MILLI., .METRE. ) );
#7571=AXIS2_PLACEMENT_3D ( 'NONE', #8801, #10620, #1239 ) ;
#7572=VERTEX_POINT ( 'NONE', #6797 ) ;
#7579=CARTESIAN_POINT ( 'NONE',  ( 2.262820851736500494, 10.00000000000000355, -9.633606397919622921 ) ) ;
#7580=AXIS2_PLACEMENT_3D ( 'NONE', #10708, #8111, #4144 ) ;
#7583=DIRECTION ( 'NONE',  ( 0.2499999999999950318, 0.8660254037844380415, 0.4330127018922235171 ) ) ;
#7586=EDGE_LOOP ( 'NONE', ( #10867, #2720, #9197 ) ) ;
#7591=VECTOR ( 'NONE', #2674, 1000.000000000000000 ) ;
#7593=ORIENTED_EDGE ( 'NONE', *, *, #3909, .T. ) ;
#7594=EDGE_CURVE ( 'NONE', #3717, #10548, #680, .T. ) ;
#7599=DIRECTION ( 'NONE',  ( 0.4330127018922191318, -0.8660254037844380415, 0.2500000000000026090 ) ) ;
#7600=ADVANCED_FACE ( 'NONE', ( #5962, #3343 ), #9206, .T. ) ;
#7603=CARTESIAN_POINT ( 'NONE',  ( 0.5000000000000000000, 10.00000000000000355, -6.982120021884467675 ) ) ;
#7606=CARTESIAN_POINT ( 'NONE',  ( 0.000000000000000000, 10.00000000000000355, 0.000000000000000000 ) ) ;
#7607=ORIENTED_EDGE ( 'NONE', *, *, #10696, .F. ) ;
#7608=PLANE ( 'NONE',  #7078 ) ;
#7614=AXIS2_PLACEMENT_3D ( 'NONE', #6592, #9171, #617 ) ;
#7616=AXIS2_PLACEMENT_3D ( 'NONE', #5030, #8378, #4187 ) ;
#7632=ORIENTED_EDGE ( 'NONE', *, *, #1478, .F. ) ;
#7633=VECTOR ( 'NONE', #6116, 1000.000000000000000 ) ;
#7635=CARTESIAN_POINT ( 'NONE',  ( 0.000000000000000000, 10.00000000000000355, 0.000000000000000000 ) ) ;
#7639=CIRCLE ( 'NONE', #4831, 6.999999999999997335 ) ;
#7641=AXIS2_PLACEMENT_3D ( 'NONE', #8374, #816, #5899 ) ;
#7653=CIRCLE ( 'NONE', #6428, 4.500000000000000888 ) ;
#7658=CARTESIAN_POINT ( 'NONE',  ( 6.994037468151970138, 19.34316356887877220, 0.3335819196118934293 ) ) ;
#7666=DIRECTION ( 'NONE',  ( 0.7559289460184543952, -0.000000000000000000, 0.6546536707079771977 ) ) ;
#7669=CARTESIAN_POINT ( 'NONE',  ( 0.000000000000000000, 10.00000000000000355, 0.000000000000000000 ) ) ;
#7674=CARTESIAN_POINT ( 'NONE',  ( 0.000000000000000000, 10.00000000000000355, 0.000000000000000000 ) ) ;
#7681=ORIENTED_EDGE ( 'NONE', *, *, #567, .F. ) ;
#7683=LINE ( 'NONE', #1776, #9333 ) ;
#7686=DIRECTION ( 'NONE',  ( -0.000000000000000000, -1.000000000000000000, -0.000000000000000000 ) ) ;
#7694=ORIENTED_EDGE ( 'NONE', *, *, #8689, .T. ) ;
#7701=DIRECTION ( 'NONE',  ( -0.4330127018922226290, -0.8660254037844380415, 0.2499999999999965028 ) ) ;
#7707=VERTEX_POINT ( 'NONE', #8670 ) ;
#7711=( GEOMETRIC_REPRESENTATION_CONTEXT ( 3 ) GLOBAL_UNCERTAINTY_ASSIGNED_CONTEXT ( ( #9897 ) ) GLOBAL_UNIT_ASSIGNED_CONTEXT ( ( #7566, #3186, #667 ) ) REPRESENTATION_CONTEXT ( 'NONE', 'WORKASPACE' ) );
#7714=CARTESIAN_POINT ( 'NONE',  ( 3.355508642977448552, 19.66631150450993104, 6.145599950363612507 ) ) ;
#7715=DIRECTION ( 'NONE',  ( 0.000000000000000000, 1.000000000000000000, 0.000000000000000000 ) ) ;
#7717=DIRECTION ( 'NONE',  ( -0.000000000000000000, -1.000000000000000000, -0.000000000000000000 ) ) ;
#7719=ORIENTED_EDGE ( 'NONE', *, *, #5262, .F. ) ;
#7721=VERTEX_POINT ( 'NONE', #9611 ) ;
#7726=DIRECTION ( 'NONE',  ( -0.5000000000000009992, 0.8660254037844380415, -1.745740669421570228E-15 ) ) ;
#7730=DIRECTION ( 'NONE',  ( 0.000000000000000000, -1.000000000000000000, 0.000000000000000000 ) ) ;
#7734=EDGE_CURVE ( 'NONE', #10248, #1133, #9063, .T. ) ;
#7737=VECTOR ( 'NONE', #9518, 1000.000000000000000 ) ;
#7740=ORIENTED_EDGE ( 'NONE', *, *, #10789, .F. ) ;
#7742=EDGE_CURVE ( 'NONE', #3157, #6934, #1935, .T. ) ;
#7749=EDGE_CURVE ( 'NONE', #10609, #2933, #3747, .T. ) ;
#7757=EDGE_CURVE ( 'NONE', #9309, #7572, #2743, .T. ) ;
#7758=ORIENTED_EDGE ( 'NONE', *, *, #3199, .F. ) ;
#7760=CARTESIAN_POINT ( 'NONE',  ( 6.296693311223917178, 19.03096903053430822, -3.058047309049999996 ) ) ;
#7761=DIRECTION ( 'NONE',  ( -1.000000000000000000, 0.000000000000000000, 0.000000000000000000 ) ) ;
#7766=VERTEX_POINT ( 'NONE', #2899 ) ;
#7768=ORIENTED_EDGE ( 'NONE', *, *, #4019, .F. ) ;
#7770=CARTESIAN_POINT ( 'NONE',  ( -5.446152422706653340, 10.00000000000000355, 2.566987298107729742 ) ) ;
#7776=CARTESIAN_POINT ( 'NONE',  ( -0.5000000000000000000, 19.03096903053430822, -6.982120021884467675 ) ) ;
#7784=VERTEX_POINT ( 'NONE', #3520 ) ;
#7785=AXIS2_PLACEMENT_3D ( 'NONE', #4738, #2230, #1403 ) ;
#7786=PLANE ( 'NONE',  #10749 ) ;
#7800=EDGE_LOOP ( 'NONE', ( #5099, #6519, #4851, #1183 ) ) ;
#7805=PLANE ( 'NONE',  #5449 ) ;
#7810=EDGE_CURVE ( 'NONE', #10901, #5101, #7847, .T. ) ;
#7811=LINE ( 'NONE', #4389, #8617 ) ;
#7819=CARTESIAN_POINT ( 'NONE',  ( 3.500000000000004885, 20.00000000000000355, -6.062177826491062405 ) ) ;
#7828=EDGE_CURVE ( 'NONE', #2551, #6450, #8723, .T. ) ;
#7829=( BOUNDED_CURVE ( )  B_SPLINE_CURVE ( 3, ( #7529, #78, #9959, #5762 ),
 .UNSPECIFIED., .F., .F. ) 
 B_SPLINE_CURVE_WITH_KNOTS ( ( 4, 4 ),
 ( 3.927175151554406884, 3.998664601439927857 ),
 .UNSPECIFIED. ) 
 CURVE ( )  GEOMETRIC_REPRESENTATION_ITEM ( )  RATIONAL_B_SPLINE_CURVE ( ( 1.000000000000000000, 0.9995741502243209453, 0.9995741502243209453, 1.000000000000000000 ) ) 
 REPRESENTATION_ITEM ( '' )  );
#7836=LINE ( 'NONE', #423, #2705 ) ;
#7845=VERTEX_POINT ( 'NONE', #10697 ) ;
#7847=CIRCLE ( 'NONE', #9939, 6.999999999999997335 ) ;
#7852=FACE_OUTER_BOUND ( 'NONE', #3346, .T. ) ;
#7854=CARTESIAN_POINT ( 'NONE',  ( 2.857142857142858983, 10.00000000000000355, 9.474358296526935064 ) ) ;
#7856=LINE ( 'NONE', #4498, #4577 ) ;
#7867=EDGE_LOOP ( 'NONE', ( #4805, #4653 ) ) ;
#7871=ADVANCED_FACE ( 'NONE', ( #5623 ), #592, .F. ) ;
#7881=DIRECTION ( 'NONE',  ( -0.9819805060619644088, -0.000000000000000000, -0.1889822365046201491 ) ) ;
#7892=DIRECTION ( 'NONE',  ( 0.000000000000000000, 1.000000000000000000, 0.000000000000000000 ) ) ;
#7897=VERTEX_POINT ( 'NONE', #3854 ) ;
#7898=EDGE_CURVE ( 'NONE', #10325, #10901, #531, .T. ) ;
#7903=DIRECTION ( 'NONE',  ( 0.000000000000000000, 0.000000000000000000, 1.000000000000000000 ) ) ;
#7904=EDGE_CURVE ( 'NONE', #3864, #5936, #7653, .T. ) ;
#7905=DIRECTION ( 'NONE',  ( -0.000000000000000000, -1.000000000000000000, -0.000000000000000000 ) ) ;
#7908=ORIENTED_EDGE ( 'NONE', *, *, #1213, .F. ) ;
#7911=DIRECTION ( 'NONE',  ( 0.8660254037844450359, 0.000000000000000000, -0.4999999999999888978 ) ) ;
#7913=ORIENTED_EDGE ( 'NONE', *, *, #4702, .F. ) ;
#7914=CARTESIAN_POINT ( 'NONE',  ( 0.000000000000000000, 10.00000000000000355, 0.000000000000000000 ) ) ;
#7915=FACE_OUTER_BOUND ( 'NONE', #6485, .T. ) ;
#7920=LINE ( 'NONE', #10513, #1758 ) ;
#7934=CARTESIAN_POINT ( 'NONE',  ( -5.890223162633825282, 19.34316356887879707, -3.785909150703112402 ) ) ;
#7947=DIRECTION ( 'NONE',  ( 0.000000000000000000, 0.000000000000000000, -1.000000000000000000 ) ) ;
#7948=CIRCLE ( 'NONE', #1071, 12.77350269189627063 ) ;
#7949=VECTOR ( 'NONE', #10109, 1000.000000000000114 ) ;
#7950=CYLINDRICAL_SURFACE ( 'NONE', #2168, 6.999999999999997335 ) ;
#7953=EDGE_CURVE ( 'NONE', #2787, #8771, #2949, .T. ) ;
#7965=DIRECTION ( 'NONE',  ( 0.000000000000000000, 0.000000000000000000, -1.000000000000000000 ) ) ;
#7969=VECTOR ( 'NONE', #6363, 1000.000000000000000 ) ;
#7976=CARTESIAN_POINT ( 'NONE',  ( 6.296693311223896750, 10.00000000000000355, 3.058047309050043960 ) ) ;
#7981=AXIS2_PLACEMENT_3D ( 'NONE', #6296, #10647, #3852 ) ;
#7984=VECTOR ( 'NONE', #5709, 1000.000000000000114 ) ;
#7989=CARTESIAN_POINT ( 'NONE',  ( 5.437177826491049082, 19.75000000000000355, 3.716506350946132020 ) ) ;
#7990=VECTOR ( 'NONE', #817, 1000.000000000000114 ) ;
#7996=AXIS2_PLACEMENT_3D ( 'NONE', #8997, #7505, #10666 ) ;
#8003=DIRECTION ( 'NONE',  ( 0.6123724356957986892, -0.3535533905932728427, -0.7071067811865445751 ) ) ;
#8006=AXIS2_PLACEMENT_3D ( 'NONE', #472, #6490, #8972 ) ;
#8012=DIRECTION ( 'NONE',  ( -0.7071067811865470176, 0.3535533905932748411, 0.6123724356957946924 ) ) ;
#8015=CARTESIAN_POINT ( 'NONE',  ( -5.937177826491102373, 19.75000000000001066, 2.850480947161618595 ) ) ;
#8018=DIRECTION ( 'NONE',  ( -0.3273268353539878217, 0.000000000000000000, 0.9449111825230682715 ) ) ;
#8019=ADVANCED_FACE ( 'NONE', ( #23 ), #10027, .T. ) ;
#8023=CARTESIAN_POINT ( 'NONE',  ( -0.1668442477450440553, 19.66631150450991328, -6.999999999999995559 ) ) ;
#8026=VERTEX_POINT ( 'NONE', #2554 ) ;
#8030=PRODUCT_DEFINITION_CONTEXT ( 'detailed design', #673, 'design' ) ;
#8031=CARTESIAN_POINT ( 'NONE',  ( -6.305607966083712768, 7.781088913245557848, -11.92163336986838473 ) ) ;
#8041=CARTESIAN_POINT ( 'NONE',  ( 5.978755702618532730, 19.66631150450991328, 3.644491357022537237 ) ) ;
#8048=CARTESIAN_POINT ( 'NONE',  ( 6.982120021884469452, 10.00000000000000355, -0.4999999999999756306 ) ) ;
#8050=FACE_OUTER_BOUND ( 'NONE', #6953, .T. ) ;
#8058=ORIENTED_EDGE ( 'NONE', *, *, #4211, .T. ) ;
#8062=EDGE_CURVE ( 'NONE', #8354, #7707, #1447, .T. ) ;
#8064=EDGE_CURVE ( 'NONE', #9935, #6450, #4794, .T. ) ;
#8066=AXIS2_PLACEMENT_3D ( 'NONE', #5525, #8012, #6416 ) ;
#8068=DIRECTION ( 'NONE',  ( -0.3273268353539845466, -0.000000000000000000, -0.9449111825230696038 ) ) ;
#8072=ORIENTED_EDGE ( 'NONE', *, *, #9720, .F. ) ;
#8076=DIRECTION ( 'NONE',  ( -0.4330127018922172999, -0.8660254037844380415, -0.2500000000000055511 ) ) ;
#8083=ORIENTED_EDGE ( 'NONE', *, *, #1166, .F. ) ;
#8085=ADVANCED_FACE ( 'NONE', ( #4179 ), #6008, .F. ) ;
#8093=ORIENTED_EDGE ( 'NONE', *, *, #3787, .F. ) ;
#8107=CARTESIAN_POINT ( 'NONE',  ( -3.924072712834378862, 10.00000000000000355, -5.796693311223959810 ) ) ;
#8111=DIRECTION ( 'NONE',  ( -0.000000000000000000, -1.000000000000000000, -0.000000000000000000 ) ) ;
#8130=DIRECTION ( 'NONE',  ( 0.3061862178479012875, -0.3535533905932726761, 0.8838834764831834390 ) ) ;
#8131=DIRECTION ( 'NONE',  ( 0.3061862178479106134, 0.3535533905932737864, -0.8838834764831797752 ) ) ;
#8139=AXIS2_PLACEMENT_3D ( 'NONE', #3097, #6445, #9798 ) ;
#8140=ADVANCED_FACE ( 'NONE', ( #2781 ), #2671, .T. ) ;
#8141=EDGE_CURVE ( 'NONE', #620, #7707, #5247, .T. ) ;
#8144=DIRECTION ( 'NONE',  ( 0.000000000000000000, 0.000000000000000000, -1.000000000000000000 ) ) ;
#8146=LINE ( 'NONE', #6341, #10078 ) ;
#8148=LINE ( 'NONE', #9082, #6938 ) ;
#8149=EDGE_CURVE ( 'NONE', #10544, #620, #10459, .T. ) ;
#8150=CIRCLE ( 'NONE', #9907, 12.77350269189627063 ) ;
#8157=DIRECTION ( 'NONE',  ( 0.000000000000000000, -0.8660254037844380415, 0.5000000000000009992 ) ) ;
#8158=DIRECTION ( 'NONE',  ( 0.000000000000000000, 1.000000000000000000, 0.000000000000000000 ) ) ;
#8162=ADVANCED_FACE ( 'NONE', ( #10366 ), #1981, .F. ) ;
#8163=CIRCLE ( 'NONE', #947, 6.999999999999997335 ) ;
#8165=( BOUNDED_CURVE ( )  B_SPLINE_CURVE ( 3, ( #1853, #301, #1026, #10407 ),
 .UNSPECIFIED., .F., .F. ) 
 B_SPLINE_CURVE_WITH_KNOTS ( ( 4, 4 ),
 ( 2.284520705739659263, 2.356010155625180680 ),
 .UNSPECIFIED. ) 
 CURVE ( )  GEOMETRIC_REPRESENTATION_ITEM ( )  RATIONAL_B_SPLINE_CURVE ( ( 1.000000000000000000, 0.9995741502243209453, 0.9995741502243209453, 1.000000000000000000 ) ) 
 REPRESENTATION_ITEM ( '' )  );
#8171=CARTESIAN_POINT ( 'NONE',  ( 0.000000000000000000, 10.00000000000000355, 0.000000000000000000 ) ) ;
#8185=FACE_OUTER_BOUND ( 'NONE', #9993, .T. ) ;
#8186=DIRECTION ( 'NONE',  ( 0.000000000000000000, -1.000000000000000000, 0.000000000000000000 ) ) ;
#8187=DIRECTION ( 'NONE',  ( 0.4330127018922191318, -0.8660254037844380415, 0.2500000000000024980 ) ) ;
#8188=ORIENTED_EDGE ( 'NONE', *, *, #446, .T. ) ;
#8192=FACE_OUTER_BOUND ( 'NONE', #10914, .T. ) ;
#8197=DIRECTION ( 'NONE',  ( 0.000000000000000000, -1.000000000000000000, 0.000000000000000000 ) ) ;
#8203=DIRECTION ( 'NONE',  ( 0.000000000000000000, 0.000000000000000000, -1.000000000000000000 ) ) ;
#8213=PRODUCT_CONTEXT ( 'NONE', #9136, 'mechanical' ) ;
#8215=EDGE_LOOP ( 'NONE', ( #6626, #4910, #2801, #9120, #6388, #496 ) ) ;
#8221=EDGE_CURVE ( 'NONE', #2855, #6764, #7114, .T. ) ;
#8229=LINE ( 'NONE', #1552, #3010 ) ;
#8231=COLOUR_RGB ( '', 0.40784314, 0.44705882, 0.49803922) ;
#8238=FACE_OUTER_BOUND ( 'NONE', #1271, .T. ) ;
#8244=CARTESIAN_POINT ( 'NONE',  ( 0.000000000000000000, 20.00000000000000355, 0.000000000000000000 ) ) ;
#8253=CARTESIAN_POINT ( 'NONE',  ( 1.135781565508698732E-14, 10.00000000000000355, 12.77350269189627241 ) ) ;
#8257=EDGE_CURVE ( 'NONE', #3818, #417, #6407, .T. ) ;
#8258=VERTEX_POINT ( 'NONE', #7776 ) ;
#8259=DIRECTION ( 'NONE',  ( -1.000000000000000000, 0.000000000000000000, -1.047444401652940007E-14 ) ) ;
#8263=CARTESIAN_POINT ( 'NONE',  ( 6.312177826491054411, 10.00000000000000355, 3.066987298107809679 ) ) ;
#8267=DIRECTION ( 'NONE',  ( 0.1767766952966430272, -0.3535533905932737309, -0.9185586535436907063 ) ) ;
#8269=ORIENTED_EDGE ( 'NONE', *, *, #7404, .F. ) ;
#8280=FILL_AREA_STYLE_COLOUR ( '', #4300 ) ;
#8286=VECTOR ( 'NONE', #5747, 1000.000000000000114 ) ;
#8291=VERTEX_POINT ( 'NONE', #3794 ) ;
#8296=CARTESIAN_POINT ( 'NONE',  ( 1.564302918553086774E-15, 7.000000000000003553, -12.77350269189627063 ) ) ;
#8298=DIRECTION ( 'NONE',  ( 0.2500000000000009992, -0.8660254037844380415, -0.4330127018922199089 ) ) ;
#8300=ADVANCED_FACE ( 'NONE', ( #2939 ), #1402, .T. ) ;
#8303=ORIENTED_EDGE ( 'NONE', *, *, #2138, .T. ) ;
#8309=CARTESIAN_POINT ( 'NONE',  ( -6.982120021884473005, 19.03096903053431888, 0.4999999999999268363 ) ) ;
#8310=DIRECTION ( 'NONE',  ( 0.000000000000000000, 0.000000000000000000, 1.000000000000000000 ) ) ;
#8311=AXIS2_PLACEMENT_3D ( 'NONE', #9660, #62, #174 ) ;
#8316=ORIENTED_EDGE ( 'NONE', *, *, #6854, .T. ) ;
#8318=CIRCLE ( 'NONE', #3022, 6.999999999999997335 ) ;
#8319=DIRECTION ( 'NONE',  ( 0.000000000000000000, -1.000000000000000000, 0.000000000000000000 ) ) ;
#8322=EDGE_LOOP ( 'NONE', ( #3797, #9643, #10655 ) ) ;
#8326=VECTOR ( 'NONE', #1562, 1000.000000000000000 ) ;
#8327=CARTESIAN_POINT ( 'NONE',  ( -3.924072712834378862, 19.03096903053431888, -5.796693311223959810 ) ) ;
#8328=CARTESIAN_POINT ( 'NONE',  ( -6.062177826491104149, 20.00000000000000355, 3.499999999999936495 ) ) ;
#8331=ORIENTED_EDGE ( 'NONE', *, *, #1147, .T. ) ;
#8332=EDGE_CURVE ( 'NONE', #7707, #4862, #9695, .T. ) ;
#8335=EDGE_CURVE ( 'NONE', #2855, #8771, #8146, .T. ) ;
#8346=CARTESIAN_POINT ( 'NONE',  ( -6.223805082245770670, 19.34316356887881483, 3.208128317448866618 ) ) ;
#8348=CARTESIAN_POINT ( 'NONE',  ( 3.924072712834460575, 10.00000000000000355, -5.796693311223904743 ) ) ;
#8354=VERTEX_POINT ( 'NONE', #8973 ) ;
#8359=EDGE_CURVE ( 'NONE', #1133, #10248, #6390, .T. ) ;
#8361=DIRECTION ( 'NONE',  ( 0.000000000000000000, -1.000000000000000000, 0.000000000000000000 ) ) ;
#8364=CARTESIAN_POINT ( 'NONE',  ( -0.5000000000000000000, 0.000000000000000000, 0.000000000000000000 ) ) ;
#8368=ORIENTED_EDGE ( 'NONE', *, *, #4138, .F. ) ;
#8371=DIRECTION ( 'NONE',  ( 0.000000000000000000, 0.000000000000000000, 1.000000000000000000 ) ) ;
#8373=CARTESIAN_POINT ( 'NONE',  ( 0.000000000000000000, 10.00000000000000355, 0.000000000000000000 ) ) ;
#8374=CARTESIAN_POINT ( 'NONE',  ( 11.92163336986831723, 7.781088913245557848, -6.305607966083837113 ) ) ;
#8375=LINE ( 'NONE', #2616, #7990 ) ;
#8376=ORIENTED_EDGE ( 'NONE', *, *, #1434, .T. ) ;
#8377=CARTESIAN_POINT ( 'NONE',  ( -6.296693311223874545, 10.00000000000000355, -3.058047309050087925 ) ) ;
#8378=DIRECTION ( 'NONE',  ( 0.9185586535436894851, -0.3535533905932744525, 0.1767766952966480787 ) ) ;
#8396=EDGE_CURVE ( 'NONE', #4628, #2551, #1117, .T. ) ;
#8405=DIRECTION ( 'NONE',  ( 0.000000000000000000, -1.000000000000000000, 0.000000000000000000 ) ) ;
#8408=DIRECTION ( 'NONE',  ( -0.8660254037844328234, 0.000000000000000000, -0.5000000000000101030 ) ) ;
#8409=CARTESIAN_POINT ( 'NONE',  ( 0.3335819196118727237, 19.34316356887877930, 6.994037468151971026 ) ) ;
#8414=VERTEX_POINT ( 'NONE', #6491 ) ;
#8415=ORIENTED_EDGE ( 'NONE', *, *, #2418, .F. ) ;
#8416=EDGE_CURVE ( 'NONE', #8771, #4628, #4634, .T. ) ;
#8420=FACE_OUTER_BOUND ( 'NONE', #8322, .T. ) ;
#8423=DIRECTION ( 'NONE',  ( 0.000000000000000000, -0.000000000000000000, 1.000000000000000000 ) ) ;
#8428=ORIENTED_EDGE ( 'NONE', *, *, #7757, .F. ) ;
#8436=LINE ( 'NONE', #162, #3935 ) ;
#8438=ORIENTED_EDGE ( 'NONE', *, *, #9356, .T. ) ;
#8447=DIRECTION ( 'NONE',  ( 0.000000000000000000, 1.000000000000000000, 0.000000000000000000 ) ) ;
#8462=EDGE_LOOP ( 'NONE', ( #8818, #6762, #4940 ) ) ;
#8464=ADVANCED_FACE ( 'NONE', ( #5667 ), #2184, .T. ) ;
#8468=ORIENTED_EDGE ( 'NONE', *, *, #9227, .T. ) ;
#8470=EDGE_LOOP ( 'NONE', ( #4667, #3876, #7913, #6551 ) ) ;
#8476=DIRECTION ( 'NONE',  ( 0.000000000000000000, 1.000000000000000000, 0.000000000000000000 ) ) ;
#8484=EDGE_CURVE ( 'NONE', #1515, #4439, #3338, .T. ) ;
#8485=ORIENTED_EDGE ( 'NONE', *, *, #10728, .T. ) ;
#8489=CARTESIAN_POINT ( 'NONE',  ( -0.5000000000000000000, 19.03096903053429756, 6.982120021884467675 ) ) ;
#8511=ORIENTED_EDGE ( 'NONE', *, *, #9143, .T. ) ;
#8512=VERTEX_POINT ( 'NONE', #13 ) ;
#8513=VERTEX_POINT ( 'NONE', #1508 ) ;
#8518=( BOUNDED_CURVE ( )  B_SPLINE_CURVE ( 3, ( #159, #3519, #2688, #5258 ),
 .UNSPECIFIED., .F., .F. ) 
 B_SPLINE_CURVE_WITH_KNOTS ( ( 4, 4 ),
 ( 2.284520705739655710, 2.356010155625175795 ),
 .UNSPECIFIED. ) 
 CURVE ( )  GEOMETRIC_REPRESENTATION_ITEM ( )  RATIONAL_B_SPLINE_CURVE ( ( 1.000000000000000000, 0.9995741502243209453, 0.9995741502243209453, 1.000000000000000000 ) ) 
 REPRESENTATION_ITEM ( '' )  );
#8524=CARTESIAN_POINT ( 'NONE',  ( -11.92163336986836875, 7.781088913245563177, 6.305607966083758953 ) ) ;
#8527=AXIS2_PLACEMENT_3D ( 'NONE', #6625, #999, #5142 ) ;
#8529=CARTESIAN_POINT ( 'NONE',  ( -6.776463540776843431, 10.00000000000000355, 7.211537444790383056 ) ) ;
#8533=ORIENTED_EDGE ( 'NONE', *, *, #1442, .T. ) ;
#8534=DIRECTION ( 'NONE',  ( -0.8660254037844432595, 0.000000000000000000, 0.4999999999999919509 ) ) ;
#8535=PLANE ( 'NONE',  #6245 ) ;
#8569=ADVANCED_FACE ( 'NONE', ( #742 ), #5010, .T. ) ;
#8587=VERTEX_POINT ( 'NONE', #2545 ) ;
#8593=CARTESIAN_POINT ( 'NONE',  ( -6.062177826491028654, 20.00000000000000355, -3.500000000000069722 ) ) ;
#8595=CARTESIAN_POINT ( 'NONE',  ( 0.000000000000000000, 10.00000000000000355, 0.000000000000000000 ) ) ;
#8602=FACE_OUTER_BOUND ( 'NONE', #3966, .T. ) ;
#8605=ORIENTED_EDGE ( 'NONE', *, *, #9765, .F. ) ;
#8606=DIRECTION ( 'NONE',  ( 0.000000000000000000, 1.000000000000000000, 0.000000000000000000 ) ) ;
#8608=CARTESIAN_POINT ( 'NONE',  ( 6.062177826491077504, 20.00000000000000355, -3.499999999999985345 ) ) ;
#8613=ADVANCED_FACE ( 'NONE', ( #685 ), #3610, .T. ) ;
#8617=VECTOR ( 'NONE', #6875, 999.9999999999998863 ) ;
#8618=FACE_OUTER_BOUND ( 'NONE', #776, .T. ) ;
#8622=CARTESIAN_POINT ( 'NONE',  ( -0.5000000000000000000, 10.00000000000000355, 6.982120021884467675 ) ) ;
#8623=DIRECTION ( 'NONE',  ( -0.4330127018922207971, 0.8660254037844380415, 0.2499999999999995282 ) ) ;
#8647=ORIENTED_EDGE ( 'NONE', *, *, #10033, .T. ) ;
#8651=EDGE_CURVE ( 'NONE', #8512, #5101, #1854, .T. ) ;
#8657=CIRCLE ( 'NONE', #6380, 6.999999999999997335 ) ;
#8660=ORIENTED_EDGE ( 'NONE', *, *, #9085, .F. ) ;
#8663=AXIS2_PLACEMENT_3D ( 'NONE', #3496, #9476, #6279 ) ;
#8665=CARTESIAN_POINT ( 'NONE',  ( -1.745740669421566678E-15, 0.000000000000000000, 0.5000000000000000000 ) ) ;
#8666=VECTOR ( 'NONE', #3454, 1000.000000000000000 ) ;
#8668=ORIENTED_EDGE ( 'NONE', *, *, #10728, .F. ) ;
#8670=CARTESIAN_POINT ( 'NONE',  ( -6.386751345948222358, 10.00000000000000355, 11.06217782649103043 ) ) ;
#8672=DIRECTION ( 'NONE',  ( -0.000000000000000000, -1.000000000000000000, -0.000000000000000000 ) ) ;
#8673=EDGE_LOOP ( 'NONE', ( #858, #4267, #5092, #10075, #5588, #9896 ) ) ;
#8674=AXIS2_PLACEMENT_3D ( 'NONE', #7104, #2217, #4724 ) ;
#8689=EDGE_CURVE ( 'NONE', #528, #3304, #10610, .T. ) ;
#8698=CARTESIAN_POINT ( 'NONE',  ( 0.000000000000000000, 10.00000000000000355, 0.000000000000000000 ) ) ;
#8699=AXIS2_PLACEMENT_3D ( 'NONE', #7674, #222, #6137 ) ;
#8704=ORIENTED_EDGE ( 'NONE', *, *, #797, .T. ) ;
#8709=ADVANCED_FACE ( 'NONE', ( #5341 ), #6114, .F. ) ;
#8711=PLANE ( 'NONE',  #2075 ) ;
#8715=LINE ( 'NONE', #312, #9764 ) ;
#8717=CARTESIAN_POINT ( 'NONE',  ( 6.776463540776787475, 10.00000000000000355, -7.211537444790439899 ) ) ;
#8718=CARTESIAN_POINT ( 'NONE',  ( 5.999999999999996447, 10.00000000000000355, 0.5000000000000209832 ) ) ;
#8721=ORIENTED_EDGE ( 'NONE', *, *, #382, .T. ) ;
#8723=CIRCLE ( 'NONE', #7138, 6.999999999999997335 ) ;
#8746=CARTESIAN_POINT ( 'NONE',  ( 11.06217782649109260, 10.00000000000000178, -6.386751345948117553 ) ) ;
#8757=LINE ( 'NONE', #136, #3205 ) ;
#8758=ADVANCED_FACE ( 'NONE', ( #5598 ), #6325, .T. ) ;
#8770=ORIENTED_EDGE ( 'NONE', *, *, #3003, .F. ) ;
#8771=VERTEX_POINT ( 'NONE', #9014 ) ;
#8801=CARTESIAN_POINT ( 'NONE',  ( 5.237222008264700033E-15, 0.000000000000000000, -0.5000000000000000000 ) ) ;
#8805=ORIENTED_EDGE ( 'NONE', *, *, #10506, .F. ) ;
#8813=EDGE_CURVE ( 'NONE', #7572, #5713, #9373, .T. ) ;
#8816=CIRCLE ( 'NONE', #4058, 6.999999999999997335 ) ;
#8818=ORIENTED_EDGE ( 'NONE', *, *, #10797, .F. ) ;
#8819=ADVANCED_FACE ( 'NONE', ( #3088 ), #462, .T. ) ;
#8825=AXIS2_PLACEMENT_3D ( 'NONE', #165, #2633, #5150 ) ;
#8826=DIRECTION ( 'NONE',  ( -0.000000000000000000, 1.000000000000000000, -0.000000000000000000 ) ) ;
#8831=AXIS2_PLACEMENT_3D ( 'NONE', #4635, #1254, #6394 ) ;
#8836=CARTESIAN_POINT ( 'NONE',  ( 6.296693311223896750, 19.03096903053431177, 3.058047309050043960 ) ) ;
#8842=CARTESIAN_POINT ( 'NONE',  ( 0.000000000000000000, 20.00000000000000355, -6.999999999999997335 ) ) ;
#8850=DIRECTION ( 'NONE',  ( 0.000000000000000000, 0.000000000000000000, 1.000000000000000000 ) ) ;
#8859=ORIENTED_EDGE ( 'NONE', *, *, #4218, .F. ) ;
#8860=ORIENTED_EDGE ( 'NONE', *, *, #196, .F. ) ;
#8869=AXIS2_PLACEMENT_3D ( 'NONE', #8364, #7532, #9963 ) ;
#8870=DIRECTION ( 'NONE',  ( 0.000000000000000000, 1.000000000000000000, 0.000000000000000000 ) ) ;
#8874=ORIENTED_EDGE ( 'NONE', *, *, #3199, .T. ) ;
#8882=DIRECTION ( 'NONE',  ( 0.000000000000000000, 0.000000000000000000, 1.000000000000000000 ) ) ;
#8890=PLANE ( 'NONE',  #8066 ) ;
#8897=CARTESIAN_POINT ( 'NONE',  ( -0.5000000000000000000, 10.00000000000000355, -6.982120021884467675 ) ) ;
#8910=DIRECTION ( 'NONE',  ( 0.8660254037844363761, 0.000000000000000000, 0.5000000000000039968 ) ) ;
#8913=ORIENTED_EDGE ( 'NONE', *, *, #7810, .T. ) ;
#8915=CARTESIAN_POINT ( 'NONE',  ( 3.785909150703014259, 19.34316356887877575, 5.890223162633890119 ) ) ;
#8920=FACE_OUTER_BOUND ( 'NONE', #8215, .T. ) ;
#8927=DIRECTION ( 'NONE',  ( 0.5000000000000009992, 0.8660254037844380415, 5.237222008264710288E-15 ) ) ;
#8937=ORIENTED_EDGE ( 'NONE', *, *, #10774, .T. ) ;
#8941=VERTEX_POINT ( 'NONE', #8348 ) ;
#8946=ORIENTED_EDGE ( 'NONE', *, *, #4396, .F. ) ;
#8948=ORIENTED_EDGE ( 'NONE', *, *, #6061, .F. ) ;
#8957=EDGE_CURVE ( 'NONE', #3717, #1851, #5048, .T. ) ;
#8963=ORIENTED_EDGE ( 'NONE', *, *, #8813, .F. ) ;
#8965=ORIENTED_EDGE ( 'NONE', *, *, #5914, .F. ) ;
#8970=EDGE_CURVE ( 'NONE', #2933, #5713, #7402, .T. ) ;
#8972=DIRECTION ( 'NONE',  ( 0.000000000000000000, 0.000000000000000000, 1.000000000000000000 ) ) ;
#8973=CARTESIAN_POINT ( 'NONE',  ( -11.06217782649114589, 10.00000000000000355, 6.386751345948025183 ) ) ;
#8975=DIRECTION ( 'NONE',  ( 0.000000000000000000, 0.000000000000000000, 1.000000000000000000 ) ) ;
#8976=ORIENTED_EDGE ( 'NONE', *, *, #8970, .F. ) ;
#8980=EDGE_CURVE ( 'NONE', #6448, #10381, #8229, .T. ) ;
#8985=DIRECTION ( 'NONE',  ( 0.8660254037844397068, 0.000000000000000000, -0.4999999999999979461 ) ) ;
#8997=CARTESIAN_POINT ( 'NONE',  ( 0.000000000000000000, 10.00000000000000355, 0.000000000000000000 ) ) ;
#9000=VECTOR ( 'NONE', #10581, 1000.000000000000000 ) ;
#9003=( BOUNDED_CURVE ( )  B_SPLINE_CURVE ( 3, ( #8608, #1767, #9318, #3523 ),
 .UNSPECIFIED., .F., .F. ) 
 B_SPLINE_CURVE_WITH_KNOTS ( ( 4, 4 ),
 ( 2.284520705739661484, 2.356010155625182012 ),
 .UNSPECIFIED. ) 
 CURVE ( )  GEOMETRIC_REPRESENTATION_ITEM ( )  RATIONAL_B_SPLINE_CURVE ( ( 1.000000000000000000, 0.9995741502243209453, 0.9995741502243209453, 1.000000000000000000 ) ) 
 REPRESENTATION_ITEM ( '' )  );
#9010=EDGE_CURVE ( 'NONE', #8258, #2606, #2428, .T. ) ;
#9011=CARTESIAN_POINT ( 'NONE',  ( -5.796693311223863887, 10.00000000000000355, -3.924072712834521415 ) ) ;
#9014=CARTESIAN_POINT ( 'NONE',  ( 10.31217782649105352, 10.00000000000000355, 6.531088913245589822 ) ) ;
#9036=ORIENTED_EDGE ( 'NONE', *, *, #7404, .T. ) ;
#9039=VECTOR ( 'NONE', #8197, 1000.000000000000000 ) ;
#9043=CARTESIAN_POINT ( 'NONE',  ( 0.000000000000000000, 10.00000000000000355, 0.000000000000000000 ) ) ;
#9045=AXIS2_PLACEMENT_3D ( 'NONE', #5072, #21, #7541 ) ;
#9047=ADVANCED_FACE ( 'NONE', ( #3241 ), #9273, .T. ) ;
#9055=DIRECTION ( 'NONE',  ( 0.8660254037844363761, 0.000000000000000000, 0.5000000000000039968 ) ) ;
#9058=PLANE ( 'NONE',  #7996 ) ;
#9060=ORIENTED_EDGE ( 'NONE', *, *, #8257, .F. ) ;
#9063=CIRCLE ( 'NONE', #6968, 4.500000000000000888 ) ;
#9065=CARTESIAN_POINT ( 'NONE',  ( 11.06217782649104997, 10.00000000000000355, 6.386751345948187719 ) ) ;
#9077=DIRECTION ( 'NONE',  ( 0.000000000000000000, 1.000000000000000000, 0.000000000000000000 ) ) ;
#9082=CARTESIAN_POINT ( 'NONE',  ( 0.5000000000000000000, 19.74999999999999645, -6.566987298107768822 ) ) ;
#9084=VERTEX_POINT ( 'NONE', #4106 ) ;
#9085=EDGE_CURVE ( 'NONE', #3717, #417, #1109, .T. ) ;
#9087=DIRECTION ( 'NONE',  ( -0.1767766952966274840, 0.3535533905932751741, -0.9185586535436930378 ) ) ;
#9093=ORIENTED_EDGE ( 'NONE', *, *, #7742, .T. ) ;
#9096=CARTESIAN_POINT ( 'NONE',  ( -5.999999999999992895, 10.00000000000000355, -0.5000000000000628386 ) ) ;
#9102=PLANE ( 'NONE',  #10469 ) ;
#9112=CARTESIAN_POINT ( 'NONE',  ( 0.000000000000000000, 20.00000000000000355, -6.999999999999997335 ) ) ;
#9115=LINE ( 'NONE', #1551, #880 ) ;
#9119=VECTOR ( 'NONE', #6442, 1000.000000000000000 ) ;
#9120=ORIENTED_EDGE ( 'NONE', *, *, #2395, .T. ) ;
#9122=VECTOR ( 'NONE', #9426, 1000.000000000000227 ) ;
#9136=APPLICATION_CONTEXT ( 'automotive_design' ) ;
#9137=EDGE_LOOP ( 'NONE', ( #8428, #9932, #6651, #6015 ) ) ;
#9139=PLANE ( 'NONE',  #5697 ) ;
#9140=CARTESIAN_POINT ( 'NONE',  ( -6.999999999999997335, 20.00000000000000355, -7.332110811570577522E-14 ) ) ;
#9143=EDGE_CURVE ( 'NONE', #8513, #1851, #8150, .T. ) ;
#9148=ORIENTED_EDGE ( 'NONE', *, *, #1938, .T. ) ;
#9155=DIRECTION ( 'NONE',  ( 0.000000000000000000, -0.000000000000000000, 1.000000000000000000 ) ) ;
#9159=ORIENTED_EDGE ( 'NONE', *, *, #3967, .T. ) ;
#9167=ORIENTED_EDGE ( 'NONE', *, *, #8980, .T. ) ;
#9170=DIRECTION ( 'NONE',  ( 0.000000000000000000, -1.000000000000000000, 0.000000000000000000 ) ) ;
#9171=DIRECTION ( 'NONE',  ( -0.6123724356957870318, 0.3535533905932747301, -0.7071067811865536790 ) ) ;
#9172=CARTESIAN_POINT ( 'NONE',  ( -3.433012701892259155, 10.00000000000000355, 4.946152422706602714 ) ) ;
#9174=VERTEX_POINT ( 'NONE', #2045 ) ;
#9183=LINE ( 'NONE', #2755, #2689 ) ;
#9196=AXIS2_PLACEMENT_3D ( 'NONE', #10093, #874, #5788 ) ;
#9197=ORIENTED_EDGE ( 'NONE', *, *, #10181, .T. ) ;
#9201=LINE ( 'NONE', #2304, #6849 ) ;
#9205=CIRCLE ( 'NONE', #10631, 12.77350269189627063 ) ;
#9206=PLANE ( 'NONE',  #8527 ) ;
#9211=ORIENTED_EDGE ( 'NONE', *, *, #10780, .T. ) ;
#9212=AXIS2_PLACEMENT_3D ( 'NONE', #3710, #2754, #7091 ) ;
#9219=LINE ( 'NONE', #1662, #10274 ) ;
#9227=EDGE_CURVE ( 'NONE', #9763, #2965, #397, .T. ) ;
#9235=CARTESIAN_POINT ( 'NONE',  ( -11.92163336986823374, 7.781088913245559624, -6.305607966084005866 ) ) ;
#9237=DIRECTION ( 'NONE',  ( 0.5000000000000101030, 0.000000000000000000, -0.8660254037844328234 ) ) ;
#9240=CARTESIAN_POINT ( 'NONE',  ( 6.982120021884465899, 19.03096903053429401, 0.5000000000000244249 ) ) ;
#9246=CARTESIAN_POINT ( 'NONE',  ( 3.499999999999963141, 20.00000000000000355, 6.062177826491089050 ) ) ;
#9249=CARTESIAN_POINT ( 'NONE',  ( 6.982120021884465899, 10.00000000000000355, 0.5000000000000244249 ) ) ;
#9255=VERTEX_POINT ( 'NONE', #1779 ) ;
#9258=CARTESIAN_POINT ( 'NONE',  ( -6.982120021884473005, 19.03096903053431888, 0.4999999999999268363 ) ) ;
#9260=EDGE_CURVE ( 'NONE', #9521, #3157, #2664, .T. ) ;
#9261=ORIENTED_EDGE ( 'NONE', *, *, #4682, .F. ) ;
#9273=PLANE ( 'NONE',  #7614 ) ;
#9274=FACE_OUTER_BOUND ( 'NONE', #10611, .T. ) ;
#9287=DIRECTION ( 'NONE',  ( -0.000000000000000000, 1.000000000000000000, -0.000000000000000000 ) ) ;
#9288=CARTESIAN_POINT ( 'NONE',  ( 6.062177826491051746, 20.00000000000000355, 3.500000000000027089 ) ) ;
#9293=VERTEX_POINT ( 'NONE', #10748 ) ;
#9298=CARTESIAN_POINT ( 'NONE',  ( 6.580127018922133253, 10.00000000000000355, 11.12916512459891116 ) ) ;
#9309=VERTEX_POINT ( 'NONE', #2299 ) ;
#9310=VECTOR ( 'NONE', #4243, 1000.000000000000000 ) ;
#9316=CARTESIAN_POINT ( 'NONE',  ( -3.785909150702975179, 19.34316356887877930, -5.890223162633914988 ) ) ;
#9317=ORIENTED_EDGE ( 'NONE', *, *, #1008, .F. ) ;
#9318=CARTESIAN_POINT ( 'NONE',  ( 5.890223162633874132, 19.34316356887878641, -3.785909150703038240 ) ) ;
#9333=VECTOR ( 'NONE', #10166, 1000.000000000000000 ) ;
#9338=EDGE_LOOP ( 'NONE', ( #3019, #7340, #6595, #10790, #7354, #2558 ) ) ;
#9356=EDGE_CURVE ( 'NONE', #5164, #1987, #6457, .T. ) ;
#9357=ORIENTED_EDGE ( 'NONE', *, *, #5404, .F. ) ;
#9358=VERTEX_POINT ( 'NONE', #2195 ) ;
#9362=( BOUNDED_CURVE ( )  B_SPLINE_CURVE ( 3, ( #2050, #4554, #2907, #8836 ),
 .UNSPECIFIED., .F., .F. ) 
 B_SPLINE_CURVE_WITH_KNOTS ( ( 4, 4 ),
 ( 2.284520705739657487, 2.356010155625178015 ),
 .UNSPECIFIED. ) 
 CURVE ( )  GEOMETRIC_REPRESENTATION_ITEM ( )  RATIONAL_B_SPLINE_CURVE ( ( 1.000000000000000000, 0.9995741502243209453, 0.9995741502243209453, 1.000000000000000000 ) ) 
 REPRESENTATION_ITEM ( '' )  );
#9364=EDGE_CURVE ( 'NONE', #689, #9550, #9914, .T. ) ;
#9367=DIRECTION ( 'NONE',  ( 0.8660254037844450359, 0.000000000000000000, -0.4999999999999888978 ) ) ;
#9369=CARTESIAN_POINT ( 'NONE',  ( 0.000000000000000000, 10.00000000000000355, 0.000000000000000000 ) ) ;
#9373=CIRCLE ( 'NONE', #10787, 12.77350269189627063 ) ;
#9378=VECTOR ( 'NONE', #6701, 1000.000000000000114 ) ;
#9401=CIRCLE ( 'NONE', #8699, 6.999999999999997335 ) ;
#9413=FACE_OUTER_BOUND ( 'NONE', #10669, .T. ) ;
#9421=EDGE_CURVE ( 'NONE', #375, #9255, #4906, .T. ) ;
#9426=DIRECTION ( 'NONE',  ( -0.9449111825230641637, 0.000000000000000000, -0.3273268353539998121 ) ) ;
#9431=DIRECTION ( 'NONE',  ( -0.2500000000000041078, -0.8660254037844380415, 0.4330127018922181881 ) ) ;
#9437=ADVANCED_FACE ( 'NONE', ( #3972 ), #6616, .F. ) ;
#9442=DIRECTION ( 'NONE',  ( 1.000000000000000000, 0.000000000000000000, 3.491481338843133355E-15 ) ) ;
#9450=ADVANCED_FACE ( 'NONE', ( #8050 ), #4353, .T. ) ;
#9451=EDGE_CURVE ( 'NONE', #6293, #9491, #8375, .T. ) ;
#9461=CARTESIAN_POINT ( 'NONE',  ( 0.000000000000000000, 10.00000000000000355, 0.000000000000000000 ) ) ;
#9465=ORIENTED_EDGE ( 'NONE', *, *, #4841, .F. ) ;
#9472=ORIENTED_EDGE ( 'NONE', *, *, #8149, .F. ) ;
#9474=CARTESIAN_POINT ( 'NONE',  ( -6.062177826491031318, 20.00000000000000355, -3.500000000000064393 ) ) ;
#9475=DIRECTION ( 'NONE',  ( -0.5000000000000039968, 0.000000000000000000, 0.8660254037844363761 ) ) ;
#9476=DIRECTION ( 'NONE',  ( 0.000000000000000000, -1.000000000000000000, 0.000000000000000000 ) ) ;
#9483=STYLED_ITEM ( 'NONE', ( #1548 ), #10206 ) ;
#9486=DIRECTION ( 'NONE',  ( 0.000000000000000000, 1.000000000000000000, 0.000000000000000000 ) ) ;
#9487=PLANE ( 'NONE',  #9752 ) ;
#9491=VERTEX_POINT ( 'NONE', #3328 ) ;
#9496=PLANE ( 'NONE',  #328 ) ;
#9497=ADVANCED_FACE ( 'NONE', ( #1694 ), #3511, .F. ) ;
#9504=CARTESIAN_POINT ( 'NONE',  ( 3.924072712834419718, 10.00000000000000355, 5.796693311223933165 ) ) ;
#9507=EDGE_CURVE ( 'NONE', #10609, #5553, #5026, .T. ) ;
#9518=DIRECTION ( 'NONE',  ( -0.000000000000000000, -1.000000000000000000, -0.000000000000000000 ) ) ;
#9521=VERTEX_POINT ( 'NONE', #10085 ) ;
#9523=ORIENTED_EDGE ( 'NONE', *, *, #9451, .F. ) ;
#9535=LINE ( 'NONE', #6229, #9747 ) ;
#9538=FACE_OUTER_BOUND ( 'NONE', #3401, .T. ) ;
#9544=LINE ( 'NONE', #8717, #762 ) ;
#9545=CARTESIAN_POINT ( 'NONE',  ( -11.26313972081434223, 10.00000000000000355, -6.348076211353453679 ) ) ;
#9546=FACE_OUTER_BOUND ( 'NONE', #7800, .T. ) ;
#9550=VERTEX_POINT ( 'NONE', #9249 ) ;
#9551=EDGE_LOOP ( 'NONE', ( #7108, #1556, #1444 ) ) ;
#9556=LINE ( 'NONE', #9657, #10046 ) ;
#9564=LINE ( 'NONE', #1279, #7969 ) ;
#9567=DIRECTION ( 'NONE',  ( 0.000000000000000000, 0.000000000000000000, 1.000000000000000000 ) ) ;
#9571=ORIENTED_EDGE ( 'NONE', *, *, #6271, .T. ) ;
#9572=ORIENTED_EDGE ( 'NONE', *, *, #2029, .F. ) ;
#9574=CIRCLE ( 'NONE', #4812, 12.77350269189627063 ) ;
#9589=LINE ( 'NONE', #10356, #4433 ) ;
#9591=VECTOR ( 'NONE', #7881, 1000.000000000000227 ) ;
#9593=VERTEX_POINT ( 'NONE', #3686 ) ;
#9595=DIRECTION ( 'NONE',  ( 0.000000000000000000, 0.000000000000000000, -1.000000000000000000 ) ) ;
#9597=ADVANCED_FACE ( 'NONE', ( #9546 ), #426, .T. ) ;
#9604=FACE_OUTER_BOUND ( 'NONE', #1196, .T. ) ;
#9608=LINE ( 'NONE', #5559, #6153 ) ;
#9611=CARTESIAN_POINT ( 'NONE',  ( 0.000000000000000000, 20.00000000000000355, -2.149999999999999911 ) ) ;
#9618=PLANE ( 'NONE',  #320 ) ;
#9622=DIRECTION ( 'NONE',  ( 0.000000000000000000, 1.000000000000000000, 0.000000000000000000 ) ) ;
#9629=CARTESIAN_POINT ( 'NONE',  ( 0.000000000000000000, 20.00000000000000355, 6.999999999999997335 ) ) ;
#9633=ADVANCED_FACE ( 'NONE', ( #9604 ), #5250, .F. ) ;
#9634=EDGE_CURVE ( 'NONE', #10381, #4561, #8318, .T. ) ;
#9635=CARTESIAN_POINT ( 'NONE',  ( -11.12916512459892893, 10.00000000000000355, 6.580127018922093285 ) ) ;
#9636=LINE ( 'NONE', #10566, #10418 ) ;
#9637=ADVANCED_FACE ( 'NONE', ( #1102 ), #7118, .F. ) ;
#9643=ORIENTED_EDGE ( 'NONE', *, *, #3435, .T. ) ;
#9649=DIRECTION ( 'NONE',  ( -0.000000000000000000, -1.000000000000000000, -0.000000000000000000 ) ) ;
#9650=CARTESIAN_POINT ( 'NONE',  ( 0.5000000000000000000, 10.00000000000000355, 6.982120021884467675 ) ) ;
#9657=CARTESIAN_POINT ( 'NONE',  ( 0.5000000000000000000, 10.00000000000000355, 6.999999999999997335 ) ) ;
#9660=CARTESIAN_POINT ( 'NONE',  ( 0.000000000000000000, 10.00000000000000355, 0.000000000000000000 ) ) ;
#9665=CYLINDRICAL_SURFACE ( 'NONE', #3162, 6.999999999999997335 ) ;
#9670=DIRECTION ( 'NONE',  ( -0.000000000000000000, 1.000000000000000000, -0.000000000000000000 ) ) ;
#9673=ORIENTED_EDGE ( 'NONE', *, *, #6458, .T. ) ;
#9674=VECTOR ( 'NONE', #7103, 1000.000000000000114 ) ;
#9677=ORIENTED_EDGE ( 'NONE', *, *, #10167, .T. ) ;
#9680=VECTOR ( 'NONE', #1644, 1000.000000000000000 ) ;
#9681=CARTESIAN_POINT ( 'NONE',  ( 6.348076211353333775, 10.00000000000000355, -11.26313972081440618 ) ) ;
#9686=CARTESIAN_POINT ( 'NONE',  ( 3.499999999999996447, 20.00000000000000355, -6.062177826491068622 ) ) ;
#9687=CARTESIAN_POINT ( 'NONE',  ( 0.000000000000000000, 10.00000000000000355, 0.000000000000000000 ) ) ;
#9695=LINE ( 'NONE', #473, #9913 ) ;
#9701=CIRCLE ( 'NONE', #2454, 6.999999999999997335 ) ;
#9702=EDGE_CURVE ( 'NONE', #5192, #7897, #8148, .T. ) ;
#9713=ORIENTED_EDGE ( 'NONE', *, *, #10657, .T. ) ;
#9720=EDGE_CURVE ( 'NONE', #5566, #824, #7261, .T. ) ;
#9723=CARTESIAN_POINT ( 'NONE',  ( 6.999999999999997335, 20.00000000000000355, 2.444036937190192402E-14 ) ) ;
#9734=PLANE ( 'NONE',  #7571 ) ;
#9741=AXIS2_PLACEMENT_3D ( 'NONE', #370, #2675, #5360 ) ;
#9747=VECTOR ( 'NONE', #10309, 1000.000000000000000 ) ;
#9750=AXIS2_PLACEMENT_3D ( 'NONE', #447, #9622, #1949 ) ;
#9752=AXIS2_PLACEMENT_3D ( 'NONE', #7011, #7892, #3683 ) ;
#9753=ADVANCED_FACE ( 'NONE', ( #8920 ), #4791, .T. ) ;
#9756=CARTESIAN_POINT ( 'NONE',  ( 12.19615242270662847, 10.00000000000000355, 0.5000000000000426326 ) ) ;
#9762=AXIS2_PLACEMENT_3D ( 'NONE', #1637, #6837, #8310 ) ;
#9763=VERTEX_POINT ( 'NONE', #2996 ) ;
#9764=VECTOR ( 'NONE', #7113, 1000.000000000000114 ) ;
#9765=EDGE_CURVE ( 'NONE', #5101, #1433, #10691, .T. ) ;
#9766=EDGE_LOOP ( 'NONE', ( #3988, #8438, #9211, #6346, #9677, #1480 ) ) ;
#9775=( BOUNDED_CURVE ( )  B_SPLINE_CURVE ( 3, ( #6501, #5676, #639, #5731 ),
 .UNSPECIFIED., .F., .F. ) 
 B_SPLINE_CURVE_WITH_KNOTS ( ( 4, 4 ),
 ( 3.927175151554401111, 3.998664601439922084 ),
 .UNSPECIFIED. ) 
 CURVE ( )  GEOMETRIC_REPRESENTATION_ITEM ( )  RATIONAL_B_SPLINE_CURVE ( ( 1.000000000000000000, 0.9995741502243209453, 0.9995741502243209453, 1.000000000000000000 ) ) 
 REPRESENTATION_ITEM ( '' )  );
#9777=ORIENTED_EDGE ( 'NONE', *, *, #1938, .F. ) ;
#9784=CARTESIAN_POINT ( 'NONE',  ( -6.999999999999997335, 20.00000000000000355, -7.332110811570577522E-14 ) ) ;
#9785=CARTESIAN_POINT ( 'NONE',  ( 5.796693311223893197, 10.00000000000000355, 3.924072712834480559 ) ) ;
#9787=DIRECTION ( 'NONE',  ( -0.4330127018922207971, 0.8660254037844380415, 0.2499999999999995282 ) ) ;
#9790=ORIENTED_EDGE ( 'NONE', *, *, #1928, .F. ) ;
#9792=ORIENTED_EDGE ( 'NONE', *, *, #10592, .T. ) ;
#9798=DIRECTION ( 'NONE',  ( 0.000000000000000000, 0.000000000000000000, 1.000000000000000000 ) ) ;
#9802=ORIENTED_EDGE ( 'NONE', *, *, #6854, .F. ) ;
#9806=CARTESIAN_POINT ( 'NONE',  ( -6.566987298107773263, 19.75000000000000355, -0.5000000000000687228 ) ) ;
#9810=EDGE_CURVE ( 'NONE', #4041, #9293, #8163, .T. ) ;
#9824=ORIENTED_EDGE ( 'NONE', *, *, #3348, .F. ) ;
#9827=ADVANCED_FACE ( 'NONE', ( #10188 ), #805, .T. ) ;
#9830=AXIS2_PLACEMENT_3D ( 'NONE', #2834, #6233, #9595 ) ;
#9833=CARTESIAN_POINT ( 'NONE',  ( -6.312177826491033095, 10.00000000000000355, -3.066987298107852755 ) ) ;
#9835=LINE ( 'NONE', #9635, #9674 ) ;
#9836=PLANE ( 'NONE',  #7079 ) ;
#9840=AXIS2_PLACEMENT_3D ( 'NONE', #10011, #9077, #5719 ) ;
#9846=CARTESIAN_POINT ( 'NONE',  ( 0.000000000000000000, 7.000000000000003553, 0.000000000000000000 ) ) ;
#9852=ORIENTED_EDGE ( 'NONE', *, *, #8062, .T. ) ;
#9853=ORIENTED_EDGE ( 'NONE', *, *, #3632, .F. ) ;
#9854=ORIENTED_EDGE ( 'NONE', *, *, #8484, .T. ) ;
#9860=CARTESIAN_POINT ( 'NONE',  ( 0.000000000000000000, 7.000000000000003553, 0.000000000000000000 ) ) ;
#9863=AXIS2_PLACEMENT_3D ( 'NONE', #4938, #7466, #1670 ) ;
#9864=ORIENTED_EDGE ( 'NONE', *, *, #2873, .F. ) ;
#9878=CIRCLE ( 'NONE', #10599, 2.149999999999999911 ) ;
#9883=VERTEX_POINT ( 'NONE', #4123 ) ;
#9884=CARTESIAN_POINT ( 'NONE',  ( -3.499999999999921840, 20.00000000000000355, -6.062177826491114807 ) ) ;
#9889=CARTESIAN_POINT ( 'NONE',  ( 0.000000000000000000, 20.00000000000000355, 0.000000000000000000 ) ) ;
#9896=ORIENTED_EDGE ( 'NONE', *, *, #7742, .F. ) ;
#9897=UNCERTAINTY_MEASURE_WITH_UNIT (LENGTH_MEASURE( 1.000000000000000082E-05 ), #7566, 'distance_accuracy_value', 'NONE');
#9898=ADVANCED_FACE ( 'NONE', ( #854 ), #4953, .F. ) ;
#9899=AXIS2_PLACEMENT_3D ( 'NONE', #5561, #1460, #4737 ) ;
#9906=DIRECTION ( 'NONE',  ( 0.8660254037844397068, 0.000000000000000000, -0.4999999999999979461 ) ) ;
#9907=AXIS2_PLACEMENT_3D ( 'NONE', #2582, #10290, #2901 ) ;
#9908=ORIENTED_EDGE ( 'NONE', *, *, #1380, .F. ) ;
#9909=ADVANCED_FACE ( 'NONE', ( #7482 ), #3374, .F. ) ;
#9913=VECTOR ( 'NONE', #6393, 1000.000000000000114 ) ;
#9914=CIRCLE ( 'NONE', #7116, 6.999999999999997335 ) ;
#9919=CARTESIAN_POINT ( 'NONE',  ( 0.000000000000000000, 10.00000000000000355, 0.000000000000000000 ) ) ;
#9921=AXIS2_PLACEMENT_3D ( 'NONE', #5035, #827, #4146 ) ;
#9926=DIRECTION ( 'NONE',  ( 0.000000000000000000, -1.000000000000000000, 0.000000000000000000 ) ) ;
#9932=ORIENTED_EDGE ( 'NONE', *, *, #10533, .F. ) ;
#9933=PLANE ( 'NONE',  #9921 ) ;
#9935=VERTEX_POINT ( 'NONE', #9240 ) ;
#9939=AXIS2_PLACEMENT_3D ( 'NONE', #6918, #2690, #6088 ) ;
#9945=SURFACE_STYLE_FILL_AREA ( #5807 ) ;
#9946=CARTESIAN_POINT ( 'NONE',  ( -6.062177826491100596, 20.00000000000000355, 3.499999999999942712 ) ) ;
#9959=CARTESIAN_POINT ( 'NONE',  ( 3.644491357022514588, 19.66631150450990262, -5.978755702618546053 ) ) ;
#9963=DIRECTION ( 'NONE',  ( -0.000000000000000000, 0.000000000000000000, -1.000000000000000000 ) ) ;
#9993=EDGE_LOOP ( 'NONE', ( #3859, #6191, #7681, #1260 ) ) ;
#9996=( NAMED_UNIT ( * ) SI_UNIT ( $, .STERADIAN. ) SOLID_ANGLE_UNIT ( ) );
#10010=DIRECTION ( 'NONE',  ( -0.4999999999999888423, 0.000000000000000000, -0.8660254037844449249 ) ) ;
#10011=CARTESIAN_POINT ( 'NONE',  ( 0.000000000000000000, 20.00000000000000355, 0.000000000000000000 ) ) ;
#10014=LINE ( 'NONE', #4951, #10278 ) ;
#10019=EDGE_CURVE ( 'NONE', #2423, #4873, #7000, .T. ) ;
#10020=VERTEX_POINT ( 'NONE', #6056 ) ;
#10024=EDGE_CURVE ( 'NONE', #5725, #3304, #9535, .T. ) ;
#10027=CYLINDRICAL_SURFACE ( 'NONE', #9762, 6.999999999999997335 ) ;
#10028=LINE ( 'NONE', #9806, #5198 ) ;
#10030=EDGE_CURVE ( 'NONE', #8026, #7707, #5344, .T. ) ;
#10033=EDGE_CURVE ( 'NONE', #9593, #8354, #10245, .T. ) ;
#10035=LINE ( 'NONE', #8377, #6381 ) ;
#10042=DIRECTION ( 'NONE',  ( 0.000000000000000000, -1.000000000000000000, 0.000000000000000000 ) ) ;
#10046=VECTOR ( 'NONE', #7903, 1000.000000000000000 ) ;
#10053=ORIENTED_EDGE ( 'NONE', *, *, #2748, .F. ) ;
#10054=SURFACE_STYLE_FILL_AREA ( #1665 ) ;
#10059=VECTOR ( 'NONE', #1043, 1000.000000000000114 ) ;
#10062=VERTEX_POINT ( 'NONE', #6886 ) ;
#10075=ORIENTED_EDGE ( 'NONE', *, *, #8813, .T. ) ;
#10078=VECTOR ( 'NONE', #2074, 1000.000000000000114 ) ;
#10080=CYLINDRICAL_SURFACE ( 'NONE', #9045, 12.77350269189627063 ) ;
#10082=CARTESIAN_POINT ( 'NONE',  ( 0.000000000000000000, 7.000000000000003553, 0.000000000000000000 ) ) ;
#10084=CARTESIAN_POINT ( 'NONE',  ( 3.058047309049977791, 10.00000000000000355, 6.296693311223928724 ) ) ;
#10085=CARTESIAN_POINT ( 'NONE',  ( 0.5000000000000001110, 10.00000000000000355, 6.982120021884469452 ) ) ;
#10090=CARTESIAN_POINT ( 'NONE',  ( 9.474358296526961709, 10.00000000000000355, -2.857142857142823011 ) ) ;
#10093=CARTESIAN_POINT ( 'NONE',  ( 0.000000000000000000, 10.10000000000000497, 0.000000000000000000 ) ) ;
#10098=EDGE_CURVE ( 'NONE', #4873, #1851, #8757, .T. ) ;
#10102=CARTESIAN_POINT ( 'NONE',  ( 3.924072712834459686, 10.00000000000000355, -5.796693311223905631 ) ) ;
#10109=DIRECTION ( 'NONE',  ( -0.4330127018922225179, -0.8660254037844380415, 0.2499999999999964473 ) ) ;
#10110=DIRECTION ( 'NONE',  ( 0.2500000000000041078, 0.8660254037844380415, -0.4330127018922181881 ) ) ;
#10112=ORIENTED_EDGE ( 'NONE', *, *, #1478, .T. ) ;
#10117=VECTOR ( 'NONE', #1474, 1000.000000000000000 ) ;
#10125=ORIENTED_EDGE ( 'NONE', *, *, #3770, .F. ) ;
#10130=DIRECTION ( 'NONE',  ( 0.000000000000000000, -1.000000000000000000, 0.000000000000000000 ) ) ;
#10136=EDGE_LOOP ( 'NONE', ( #4500, #9159, #10706 ) ) ;
#10141=ORIENTED_EDGE ( 'NONE', *, *, #8335, .T. ) ;
#10144=FACE_OUTER_BOUND ( 'NONE', #3102, .T. ) ;
#10149=DIRECTION ( 'NONE',  ( -0.000000000000000000, -1.000000000000000000, -0.000000000000000000 ) ) ;
#10150=DIRECTION ( 'NONE',  ( 0.000000000000000000, 0.000000000000000000, 1.000000000000000000 ) ) ;
#10157=VERTEX_POINT ( 'NONE', #1847 ) ;
#10163=CARTESIAN_POINT ( 'NONE',  ( 3.924072712834459686, 19.03096903053429756, -5.796693311223905631 ) ) ;
#10166=DIRECTION ( 'NONE',  ( -0.000000000000000000, -1.000000000000000000, -0.000000000000000000 ) ) ;
#10167=EDGE_CURVE ( 'NONE', #8513, #5192, #6048, .T. ) ;
#10181=EDGE_CURVE ( 'NONE', #4628, #2787, #1079, .T. ) ;
#10182=EDGE_LOOP ( 'NONE', ( #4223, #586, #8331, #1596, #9357, #1017 ) ) ;
#10188=FACE_OUTER_BOUND ( 'NONE', #3594, .T. ) ;
#10197=CARTESIAN_POINT ( 'NONE',  ( 6.999999999999997335, 20.00000000000000355, 2.444036937190192402E-14 ) ) ;
#10199=DIRECTION ( 'NONE',  ( 0.000000000000000000, -0.000000000000000000, 1.000000000000000000 ) ) ;
#10202=AXIS2_PLACEMENT_3D ( 'NONE', #9461, #8447, #5273 ) ;
#10206=ADVANCED_BREP_SHAPE_REPRESENTATION ( '', ( #7050, #7040 ), #1019 ) ;
#10211=DIRECTION ( 'NONE',  ( 0.000000000000000000, 0.000000000000000000, 1.000000000000000000 ) ) ;
#10217=VERTEX_POINT ( 'NONE', #1787 ) ;
#10229=VERTEX_POINT ( 'NONE', #10403 ) ;
#10245=LINE ( 'NONE', #8529, #9591 ) ;
#10248=VERTEX_POINT ( 'NONE', #2595 ) ;
#10254=DIRECTION ( 'NONE',  ( 0.000000000000000000, -0.000000000000000000, 1.000000000000000000 ) ) ;
#10257=LINE ( 'NONE', #10084, #49 ) ;
#10262=ADVANCED_FACE ( 'NONE', ( #8618 ), #2634, .F. ) ;
#10264=DIRECTION ( 'NONE',  ( 0.000000000000000000, 1.000000000000000000, 0.000000000000000000 ) ) ;
#10270=DIRECTION ( 'NONE',  ( 0.2499999999999980016, -0.8660254037844380415, 0.4330127018922217408 ) ) ;
#10271=( BOUNDED_CURVE ( )  B_SPLINE_CURVE ( 3, ( #10314, #5296, #1248, #5557 ),
 .UNSPECIFIED., .F., .F. ) 
 B_SPLINE_CURVE_WITH_KNOTS ( ( 4, 4 ),
 ( 2.284520705739661484, 2.356010155625181568 ),
 .UNSPECIFIED. ) 
 CURVE ( )  GEOMETRIC_REPRESENTATION_ITEM ( )  RATIONAL_B_SPLINE_CURVE ( ( 1.000000000000000000, 0.9995741502243209453, 0.9995741502243209453, 1.000000000000000000 ) ) 
 REPRESENTATION_ITEM ( '' )  );
#10272=CARTESIAN_POINT ( 'NONE',  ( 0.000000000000000000, 10.00000000000000355, 0.000000000000000000 ) ) ;
#10274=VECTOR ( 'NONE', #1775, 1000.000000000000000 ) ;
#10276=AXIS2_PLACEMENT_3D ( 'NONE', #10699, #2137, #5515 ) ;
#10278=VECTOR ( 'NONE', #6929, 1000.000000000000114 ) ;
#10280=CARTESIAN_POINT ( 'NONE',  ( -5.796693311223863887, 10.00000000000000355, -3.924072712834521415 ) ) ;
#10283=ORIENTED_EDGE ( 'NONE', *, *, #8396, .T. ) ;
#10289=CARTESIAN_POINT ( 'NONE',  ( 3.433012701892224516, 10.00000000000000355, -4.946152422706625806 ) ) ;
#10290=DIRECTION ( 'NONE',  ( 0.000000000000000000, 1.000000000000000000, 0.000000000000000000 ) ) ;
#10292=CIRCLE ( 'NONE', #758, 12.77350269189627063 ) ;
#10293=AXIS2_PLACEMENT_3D ( 'NONE', #10272, #2744, #10211 ) ;
#10304=DIRECTION ( 'NONE',  ( 0.4330127018922172999, 0.8660254037844380415, 0.2500000000000055511 ) ) ;
#10309=DIRECTION ( 'NONE',  ( 0.000000000000000000, -1.000000000000000000, 0.000000000000000000 ) ) ;
#10314=CARTESIAN_POINT ( 'NONE',  ( -3.500000000000049294, 20.00000000000000355, 6.062177826491040200 ) ) ;
#10319=DIRECTION ( 'NONE',  ( 0.000000000000000000, 0.000000000000000000, 1.000000000000000000 ) ) ;
#10320=FACE_OUTER_BOUND ( 'NONE', #777, .T. ) ;
#10322=CARTESIAN_POINT ( 'NONE',  ( 0.000000000000000000, 10.00000000000000355, 0.000000000000000000 ) ) ;
#10325=VERTEX_POINT ( 'NONE', #3413 ) ;
#10336=DIRECTION ( 'NONE',  ( 0.000000000000000000, 0.000000000000000000, 1.000000000000000000 ) ) ;
#10339=DIRECTION ( 'NONE',  ( 0.5000000000000009992, -0.8660254037844380415, 1.745740669421570228E-15 ) ) ;
#10349=CARTESIAN_POINT ( 'NONE',  ( 5.796693311223892309, 10.00000000000000355, 3.924072712834481447 ) ) ;
#10355=DIRECTION ( 'NONE',  ( 0.000000000000000000, 0.000000000000000000, 1.000000000000000000 ) ) ;
#10356=CARTESIAN_POINT ( 'NONE',  ( -3.924072712834500543, 10.00000000000000355, 5.796693311223878098 ) ) ;
#10357=CARTESIAN_POINT ( 'NONE',  ( -2.262820851736579986, 10.00000000000000355, 9.633606397919624698 ) ) ;
#10364=VERTEX_POINT ( 'NONE', #10163 ) ;
#10366=FACE_OUTER_BOUND ( 'NONE', #6140, .T. ) ;
#10375=CIRCLE ( 'NONE', #6314, 12.77350269189627063 ) ;
#10376=ADVANCED_FACE ( 'NONE', ( #4605 ), #8890, .T. ) ;
#10381=VERTEX_POINT ( 'NONE', #386 ) ;
#10385=DIRECTION ( 'NONE',  ( 0.000000000000000000, 0.000000000000000000, 1.000000000000000000 ) ) ;
#10390=CIRCLE ( 'NONE', #10202, 12.77350269189627063 ) ;
#10400=ORIENTED_EDGE ( 'NONE', *, *, #9143, .F. ) ;
#10403=CARTESIAN_POINT ( 'NONE',  ( -6.999999999999997335, 20.00000000000000355, -7.332110811570577522E-14 ) ) ;
#10407=CARTESIAN_POINT ( 'NONE',  ( -5.796693311223946488, 19.03096903053430466, 3.924072712834398846 ) ) ;
#10413=VERTEX_POINT ( 'NONE', #4657 ) ;
#10415=EDGE_LOOP ( 'NONE', ( #10455, #4515, #3000 ) ) ;
#10418=VECTOR ( 'NONE', #6435, 1000.000000000000114 ) ;
#10423=CARTESIAN_POINT ( 'NONE',  ( 0.000000000000000000, 10.00000000000000355, 0.000000000000000000 ) ) ;
#10428=ORIENTED_EDGE ( 'NONE', *, *, #2792, .T. ) ;
#10434=( BOUNDED_CURVE ( )  B_SPLINE_CURVE ( 3, ( #3879, #6479, #557, #9784 ),
 .UNSPECIFIED., .F., .F. ) 
 B_SPLINE_CURVE_WITH_KNOTS ( ( 4, 4 ),
 ( 3.927175151554403332, 3.998664601439923860 ),
 .UNSPECIFIED. ) 
 CURVE ( )  GEOMETRIC_REPRESENTATION_ITEM ( )  RATIONAL_B_SPLINE_CURVE ( ( 1.000000000000000000, 0.9995741502243209453, 0.9995741502243209453, 1.000000000000000000 ) ) 
 REPRESENTATION_ITEM ( '' )  );
#10440=AXIS2_PLACEMENT_3D ( 'NONE', #5500, #9649, #4007 ) ;
#10442=ADVANCED_FACE ( 'NONE', ( #3862 ), #9618, .T. ) ;
#10448=FACE_OUTER_BOUND ( 'NONE', #1032, .T. ) ;
#10449=CARTESIAN_POINT ( 'NONE',  ( 11.06217782649109260, 10.00000000000000355, -6.386751345948115777 ) ) ;
#10455=ORIENTED_EDGE ( 'NONE', *, *, #7319, .T. ) ;
#10459=CIRCLE ( 'NONE', #4284, 6.999999999999997335 ) ;
#10468=DIRECTION ( 'NONE',  ( 0.000000000000000000, 1.000000000000000000, 0.000000000000000000 ) ) ;
#10469=AXIS2_PLACEMENT_3D ( 'NONE', #10883, #3985, #9155 ) ;
#10474=ORIENTED_EDGE ( 'NONE', *, *, #8970, .T. ) ;
#10483=DIRECTION ( 'NONE',  ( 0.6123724356957902515, 0.3535533905932737309, 0.7071067811865512365 ) ) ;
#10502=ORIENTED_EDGE ( 'NONE', *, *, #478, .T. ) ;
#10506=EDGE_CURVE ( 'NONE', #10548, #2423, #5738, .T. ) ;
#10507=EDGE_CURVE ( 'NONE', #748, #9491, #2360, .T. ) ;
#10513=CARTESIAN_POINT ( 'NONE',  ( -9.633606397919589170, 10.00000000000000355, -2.262820851736602190 ) ) ;
#10517=CARTESIAN_POINT ( 'NONE',  ( 6.566987298107765270, 19.74999999999999645, 0.5000000000000228706 ) ) ;
#10524=VERTEX_POINT ( 'NONE', #3223 ) ;
#10530=CARTESIAN_POINT ( 'NONE',  ( -6.386751345947994984, 10.00000000000000355, -11.06217782649116366 ) ) ;
#10531=DIRECTION ( 'NONE',  ( 0.000000000000000000, 1.000000000000000000, 0.000000000000000000 ) ) ;
#10532=VERTEX_POINT ( 'NONE', #5842 ) ;
#10533=EDGE_CURVE ( 'NONE', #4439, #9309, #9201, .T. ) ;
#10536=FACE_OUTER_BOUND ( 'NONE', #5217, .T. ) ;
#10537=DIRECTION ( 'NONE',  ( -0.9185586535436922606, 0.3535533905932755072, 0.1767766952966313421 ) ) ;
#10539=CARTESIAN_POINT ( 'NONE',  ( 6.386751345948060710, 10.00000000000000355, 11.06217782649112458 ) ) ;
#10542=AXIS2_PLACEMENT_3D ( 'NONE', #2887, #308, #1302 ) ;
#10544=VERTEX_POINT ( 'NONE', #7279 ) ;
#10548=VERTEX_POINT ( 'NONE', #600 ) ;
#10566=CARTESIAN_POINT ( 'NONE',  ( -11.42163336986836875, 7.781088913245557848, 7.171633369868196439 ) ) ;
#10571=ORIENTED_EDGE ( 'NONE', *, *, #8141, .T. ) ;
#10572=EDGE_LOOP ( 'NONE', ( #4052, #2773, #3886, #5294, #2197, #4837 ) ) ;
#10581=DIRECTION ( 'NONE',  ( 0.000000000000000000, -1.000000000000000000, 0.000000000000000000 ) ) ;
#10589=LINE ( 'NONE', #8253, #761 ) ;
#10591=AXIS2_PLACEMENT_3D ( 'NONE', #1101, #7717, #6902 ) ;
#10592=EDGE_CURVE ( 'NONE', #10901, #6438, #938, .T. ) ;
#10599=AXIS2_PLACEMENT_3D ( 'NONE', #6793, #10149, #5841 ) ;
#10601=CARTESIAN_POINT ( 'NONE',  ( 0.4330127018922225735, 0.000000000000000000, -0.2499999999999944766 ) ) ;
#10604=DIRECTION ( 'NONE',  ( 0.4330127018922226290, 0.8660254037844380415, -0.2499999999999965028 ) ) ;
#10609=VERTEX_POINT ( 'NONE', #4186 ) ;
#10610=CIRCLE ( 'NONE', #7253, 6.999999999999997335 ) ;
#10611=EDGE_LOOP ( 'NONE', ( #4806, #1049, #18, #8468, #3483, #4459 ) ) ;
#10620=DIRECTION ( 'NONE',  ( 1.047444401652940007E-14, 0.000000000000000000, -1.000000000000000000 ) ) ;
#10623=VECTOR ( 'NONE', #2897, 1000.000000000000114 ) ;
#10631=AXIS2_PLACEMENT_3D ( 'NONE', #5721, #4889, #6603 ) ;
#10636=AXIS2_PLACEMENT_3D ( 'NONE', #5998, #5112, #5066 ) ;
#10637=DIRECTION ( 'NONE',  ( 1.000000000000000000, 0.000000000000000000, -0.000000000000000000 ) ) ;
#10644=EDGE_LOOP ( 'NONE', ( #7740, #9036, #1686, #8913, #793, #7324 ) ) ;
#10647=DIRECTION ( 'NONE',  ( -0.8660254037844415942, 0.000000000000000000, 0.4999999999999949485 ) ) ;
#10655=ORIENTED_EDGE ( 'NONE', *, *, #10592, .F. ) ;
#10656=ORIENTED_EDGE ( 'NONE', *, *, #3909, .F. ) ;
#10657=EDGE_CURVE ( 'NONE', #4468, #8291, #10375, .T. ) ;
#10662=DIRECTION ( 'NONE',  ( -0.8660254037844432595, 0.000000000000000000, 0.4999999999999919509 ) ) ;
#10666=DIRECTION ( 'NONE',  ( 0.000000000000000000, -0.000000000000000000, 1.000000000000000000 ) ) ;
#10669=EDGE_LOOP ( 'NONE', ( #1484, #2006, #8770, #2131 ) ) ;
#10677=CARTESIAN_POINT ( 'NONE',  ( 0.4330127018922172999, 0.000000000000000000, 0.2500000000000036082 ) ) ;
#10679=DIRECTION ( 'NONE',  ( -0.5000000000000039968, 0.000000000000000000, 0.8660254037844363761 ) ) ;
#10687=ORIENTED_EDGE ( 'NONE', *, *, #10774, .F. ) ;
#10691=LINE ( 'NONE', #523, #3938 ) ;
#10693=ORIENTED_EDGE ( 'NONE', *, *, #1928, .T. ) ;
#10696=EDGE_CURVE ( 'NONE', #9174, #10609, #1614, .T. ) ;
#10697=CARTESIAN_POINT ( 'NONE',  ( 6.386751345948143310, 10.00000000000000355, -11.06217782649107839 ) ) ;
#10699=CARTESIAN_POINT ( 'NONE',  ( 4.336808689942017736E-16, 20.00000000000000355, -6.999999999999997335 ) ) ;
#10706=ORIENTED_EDGE ( 'NONE', *, *, #5259, .T. ) ;
#10708=CARTESIAN_POINT ( 'NONE',  ( 0.000000000000000000, 10.10000000000000497, 0.000000000000000000 ) ) ;
#10718=AXIS2_PLACEMENT_3D ( 'NONE', #6531, #10840, #3239 ) ;
#10722=SHAPE_REPRESENTATION_RELATIONSHIP ( 'NONE' , 'NONE' ,  #6555, #10206 ) ;
#10727=VECTOR ( 'NONE', #8405, 1000.000000000000000 ) ;
#10728=EDGE_CURVE ( 'NONE', #10381, #9593, #1456, .T. ) ;
#10747=DIRECTION ( 'NONE',  ( 0.000000000000000000, 0.000000000000000000, 1.000000000000000000 ) ) ;
#10748=CARTESIAN_POINT ( 'NONE',  ( 3.500000000000004885, 20.00000000000000355, -6.062177826491062405 ) ) ;
#10749=AXIS2_PLACEMENT_3D ( 'NONE', #1107, #570, #6971 ) ;
#10751=ORIENTED_EDGE ( 'NONE', *, *, #9260, .T. ) ;
#10752=ADVANCED_FACE ( 'NONE', ( #8192 ), #9496, .T. ) ;
#10753=EDGE_CURVE ( 'NONE', #9293, #7845, #9608, .T. ) ;
#10755=AXIS2_PLACEMENT_3D ( 'NONE', #3650, #7034, #10662 ) ;
#10762=DIRECTION ( 'NONE',  ( -0.6123724356957948034, -0.3535533905932734533, 0.7071067811865474617 ) ) ;
#10764=CARTESIAN_POINT ( 'NONE',  ( -1.135781565508698732E-14, 10.00000000000000355, -12.77350269189627241 ) ) ;
#10769=ORIENTED_EDGE ( 'NONE', *, *, #10789, .T. ) ;
#10774=EDGE_CURVE ( 'NONE', #915, #10157, #7415, .T. ) ;
#10780=EDGE_CURVE ( 'NONE', #1987, #7845, #6770, .T. ) ;
#10781=VECTOR ( 'NONE', #10010, 1000.000000000000114 ) ;
#10782=( BOUNDED_CURVE ( )  B_SPLINE_CURVE ( 3, ( #7819, #1145, #6165, #3666 ),
 .UNSPECIFIED., .F., .F. ) 
 B_SPLINE_CURVE_WITH_KNOTS ( ( 4, 4 ),
 ( 2.284520705739657931, 2.356010155625176683 ),
 .UNSPECIFIED. ) 
 CURVE ( )  GEOMETRIC_REPRESENTATION_ITEM ( )  RATIONAL_B_SPLINE_CURVE ( ( 1.000000000000000000, 0.9995741502243209453, 0.9995741502243209453, 1.000000000000000000 ) ) 
 REPRESENTATION_ITEM ( '' )  );
#10787=AXIS2_PLACEMENT_3D ( 'NONE', #9687, #10468, #1388 ) ;
#10789=EDGE_CURVE ( 'NONE', #6450, #4041, #6855, .T. ) ;
#10790=ORIENTED_EDGE ( 'NONE', *, *, #1464, .T. ) ;
#10791=ORIENTED_EDGE ( 'NONE', *, *, #3632, .T. ) ;
#10796=DIRECTION ( 'NONE',  ( 0.000000000000000000, -0.000000000000000000, -1.000000000000000000 ) ) ;
#10797=EDGE_CURVE ( 'NONE', #1630, #689, #737, .T. ) ;
#10807=AXIS2_PLACEMENT_3D ( 'NONE', #2499, #8476, #8371 ) ;
#10809=ADVANCED_FACE ( 'NONE', ( #3252, #8238 ), #6650, .F. ) ;
#10811=DIRECTION ( 'NONE',  ( -0.4330127018922172999, -0.8660254037844380415, -0.2500000000000055511 ) ) ;
#10817=AXIS2_PLACEMENT_3D ( 'NONE', #115, #7686, #1068 ) ;
#10829=CARTESIAN_POINT ( 'NONE',  ( 0.5000000000000000000, 10.00000000000000355, -6.982120021884467675 ) ) ;
#10832=ORIENTED_EDGE ( 'NONE', *, *, #10030, .F. ) ;
#10837=DIRECTION ( 'NONE',  ( -0.8660254037844328234, 0.000000000000000000, -0.5000000000000101030 ) ) ;
#10840=DIRECTION ( 'NONE',  ( -0.9185586535436915945, -0.3535533905932732868, -0.1767766952966388083 ) ) ;
#10841=CARTESIAN_POINT ( 'NONE',  ( 0.000000000000000000, 20.00000000000000355, 0.000000000000000000 ) ) ;
#10848=EDGE_CURVE ( 'NONE', #8291, #8513, #2542, .T. ) ;
#10856=CARTESIAN_POINT ( 'NONE',  ( 0.2500000000000050515, 0.000000000000000000, -0.4330127018922164117 ) ) ;
#10867=ORIENTED_EDGE ( 'NONE', *, *, #7953, .T. ) ;
#10883=CARTESIAN_POINT ( 'NONE',  ( 0.000000000000000000, 10.00000000000000355, 0.000000000000000000 ) ) ;
#10886=ORIENTED_EDGE ( 'NONE', *, *, #997, .T. ) ;
#10894=FILL_AREA_STYLE_COLOUR ( '', #8231 ) ;
#10896=LINE ( 'NONE', #9011, #1743 ) ;
#10901=VERTEX_POINT ( 'NONE', #4166 ) ;
#10911=CARTESIAN_POINT ( 'NONE',  ( 0.5000000000000000000, 19.03096903053430822, 6.982120021884467675 ) ) ;
#10914=EDGE_LOOP ( 'NONE', ( #3730, #8704, #8874 ) ) ;
#10916=ORIENTED_EDGE ( 'NONE', *, *, #7828, .T. ) ;
#10923=FACE_OUTER_BOUND ( 'NONE', #1134, .T. ) ;
#10929=CARTESIAN_POINT ( 'NONE',  ( 3.716506350946109372, 19.74999999999999645, -5.437177826491055299 ) ) ;
#10932=DIRECTION ( 'NONE',  ( 0.000000000000000000, 0.000000000000000000, 1.000000000000000000 ) ) ;
ENDSEC;
END-ISO-10303-21;
